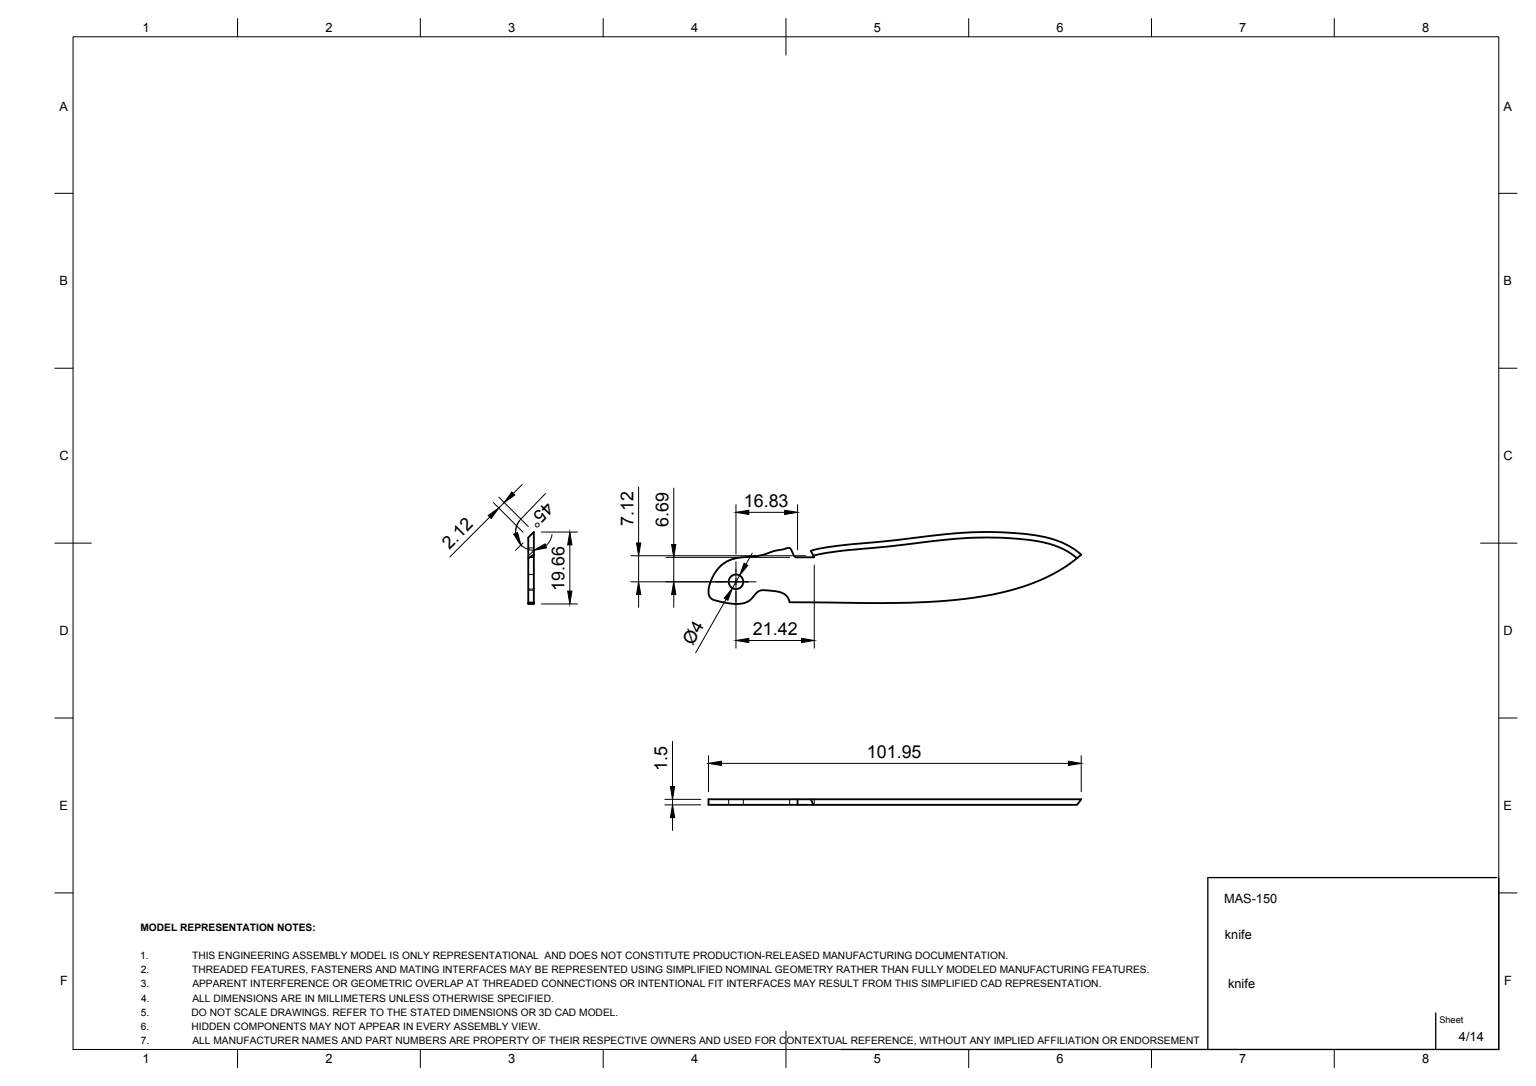
ISO-10303-21;
HEADER;
/* Generated by software containing ST-Developer
 * from STEP Tools, Inc. (www.steptools.com) 
 */

FILE_DESCRIPTION(
/* description */ ('STEP AP203'),
/* implementation_level */ '2;1');

FILE_NAME(
/* name */ 'knife.step',
/* time_stamp */ '2026-11-08T21:40:52-08:00',
/* author */ (''),
/* organization */ (''),
/* preprocessor_version */ 'ST-DEVELOPER v20.2',
/* originating_system */ 'Autodesk Translation Framework v15.17.0.0',
/* authorisation */ '');

FILE_SCHEMA (('AUTOMOTIVE_DESIGN { 1 0 10303 214 3 1 1 }'));
ENDSEC;

DATA;
#10=MECHANICAL_DESIGN_GEOMETRIC_PRESENTATION_REPRESENTATION('',(#184),#12137);
#81=B_SPLINE_CURVE_WITH_KNOTS('',3,(#2753,#2754,#2755,#2756,#2757,#2758,
#2759,#2760,#2761,#2762,#2763,#2764),.UNSPECIFIED.,.F.,.F.,(4,1,1,1,1,1,
1,1,1,4),(0.692277335272932,0.69714998216664,0.713058394872634,0.723664003343296,
0.736358399716042,0.759577826910316,0.780092040409136,0.810242072545427,
0.901462701662728,0.958125874426747),.UNSPECIFIED.);
#82=B_SPLINE_CURVE_WITH_KNOTS('',3,(#2768,#2769,#2770,#2771,#2772,#2773,
#2774,#2775,#2776,#2777,#2778,#2779),.UNSPECIFIED.,.F.,.F.,(4,1,1,1,1,1,
1,1,1,4),(0.692277335272932,0.69714998216664,0.713058394872634,0.723664003343296,
0.736358399716042,0.759577826910316,0.780092040409136,0.810242072545427,
0.901462701662728,0.958125874426747),.UNSPECIFIED.);
#83=B_SPLINE_CURVE_WITH_KNOTS('',3,(#2794,#2795,#2796,#2797,#2798,#2799),
 .UNSPECIFIED.,.F.,.F.,(4,1,1,4),(0.,0.587279823509184,0.66516934088919,
1.),.UNSPECIFIED.);
#84=B_SPLINE_CURVE_WITH_KNOTS('',3,(#2802,#2803,#2804,#2805,#2806,#2807),
 .UNSPECIFIED.,.F.,.F.,(4,1,1,4),(0.,0.587279823509184,0.66516934088919,
1.),.UNSPECIFIED.);
#85=B_SPLINE_CURVE_WITH_KNOTS('',3,(#2823,#2824,#2825,#2826,#2827,#2828,
#2829),.UNSPECIFIED.,.F.,.F.,(4,1,1,1,4),(0.,0.0866729836098282,0.459841695939614,
0.649673299675604,0.845208562818702),.UNSPECIFIED.);
#86=B_SPLINE_CURVE_WITH_KNOTS('',3,(#2831,#2832,#2833,#2834,#2835,#2836,
#2837),.UNSPECIFIED.,.F.,.F.,(4,3,4),(1.35324872955864E-8,0.631650088317911,
1.),.UNSPECIFIED.);
#87=B_SPLINE_CURVE_WITH_KNOTS('',3,(#2838,#2839,#2840,#2841,#2842,#2843,
#2844),.UNSPECIFIED.,.F.,.F.,(4,1,1,1,4),(0.,0.0866729836098282,0.459841695939614,
0.649673299675604,0.829767002127536),.UNSPECIFIED.);
#88=B_SPLINE_CURVE_WITH_KNOTS('',3,(#2847,#2848,#2849,#2850,#2851,#2852,
#2853,#2854,#2855,#2856,#2857,#2858,#2859,#2860,#2861,#2862,#2863,#2864,
#2865,#2866,#2867,#2868,#2869,#2870,#2871,#2872,#2873,#2874,#2875,#2876,
#2877,#2878,#2879,#2880,#2881,#2882,#2883,#2884,#2885,#2886,#2887,#2888,
#2889,#2890,#2891,#2892,#2893,#2894,#2895,#2896,#2897,#2898,#2899,#2900,
#2901,#2902,#2903,#2904,#2905,#2906,#2907,#2908,#2909,#2910,#2911,#2912,
#2913,#2914,#2915,#2916,#2917,#2918,#2919,#2920,#2921,#2922,#2923,#2924,
#2925,#2926,#2927,#2928,#2929,#2930,#2931,#2932,#2933,#2934,#2935,#2936,
#2937,#2938,#2939,#2940,#2941,#2942,#2943,#2944,#2945,#2946,#2947,#2948,
#2949,#2950,#2951,#2952,#2953,#2954,#2955,#2956,#2957,#2958,#2959,#2960,
#2961,#2962,#2963,#2964,#2965,#2966,#2967,#2968,#2969,#2970,#2971,#2972,
#2973,#2974,#2975,#2976,#2977,#2978,#2979,#2980,#2981,#2982,#2983,#2984,
#2985,#2986,#2987,#2988,#2989,#2990,#2991,#2992,#2993,#2994,#2995,#2996,
#2997,#2998,#2999,#3000,#3001,#3002,#3003,#3004,#3005,#3006,#3007,#3008,
#3009,#3010,#3011,#3012,#3013,#3014,#3015,#3016,#3017,#3018,#3019,#3020,
#3021,#3022,#3023,#3024,#3025,#3026,#3027,#3028,#3029,#3030,#3031,#3032,
#3033,#3034,#3035,#3036,#3037,#3038,#3039,#3040,#3041,#3042,#3043,#3044,
#3045,#3046,#3047,#3048,#3049,#3050,#3051,#3052,#3053,#3054,#3055,#3056,
#3057,#3058,#3059,#3060,#3061,#3062,#3063,#3064,#3065,#3066,#3067,#3068,
#3069,#3070,#3071,#3072,#3073,#3074,#3075,#3076,#3077,#3078,#3079,#3080,
#3081,#3082,#3083,#3084,#3085,#3086,#3087,#3088,#3089,#3090,#3091,#3092,
#3093,#3094,#3095,#3096,#3097,#3098,#3099,#3100,#3101,#3102,#3103,#3104,
#3105,#3106,#3107,#3108,#3109,#3110,#3111,#3112,#3113,#3114,#3115,#3116,
#3117,#3118,#3119,#3120,#3121,#3122,#3123,#3124,#3125,#3126,#3127,#3128,
#3129,#3130,#3131,#3132,#3133,#3134,#3135,#3136,#3137,#3138,#3139,#3140,
#3141,#3142,#3143,#3144,#3145,#3146,#3147,#3148,#3149,#3150,#3151,#3152,
#3153,#3154,#3155,#3156,#3157,#3158,#3159,#3160,#3161,#3162,#3163,#3164,
#3165,#3166,#3167,#3168,#3169,#3170,#3171,#3172,#3173,#3174,#3175,#3176,
#3177),.UNSPECIFIED.,.F.,.F.,(4,3,3,3,3,3,3,3,3,3,3,3,3,3,3,3,3,3,3,3,3,
3,3,3,3,3,3,3,3,3,3,3,3,3,3,3,3,3,3,3,3,3,3,3,3,3,3,3,3,3,3,3,3,3,3,3,3,
3,3,3,3,3,3,3,3,3,3,3,3,3,3,3,3,3,3,3,3,3,3,3,3,3,3,3,3,3,3,3,3,3,3,3,3,
3,3,3,3,3,3,3,3,3,3,3,3,3,3,3,3,3,4),(1.00000005226737E-6,0.00728562366971475,
0.0234463959847306,0.0557978953419903,0.0881792075542466,0.120578085908497,
0.199435146924132,0.250102975200852,0.332264327598246,0.378931394146745,
0.442710847956035,0.458655711408358,0.465225430544162,0.470485225689555,
0.506490301765326,0.587406978409983,0.63447750239409,0.698713581314966,
0.762996361968068,0.827238553299382,0.891353412993002,0.919885897936909,
0.925235738863892,0.927910373024815,0.929197830974231,0.93032386627772,
0.965310836068324,1.00172317218786,1.00548335276863,1.0439300169432,1.08610137935927,
1.14148474424288,1.17398141008201,1.20363917088317,1.23143564581068,1.25060619127644,
1.27597878060136,1.29260925110888,1.33079359731686,1.3485547264891,1.3496219232794,
1.35038687476659,1.36631585566134,1.43886146909154,1.48931728875302,1.51524396218266,
1.57648663203031,1.5962584262802,1.66704233666681,1.6830136697589,1.74924243686783,
1.77713875907306,1.81979916869953,1.82771178722931,1.87226124160844,1.8812062035948,
1.92683921666331,1.96328819238212,1.98151268024153,1.99062492417124,1.99518104613609,
1.99809663447909,1.99973716810094,2.11425198948044,2.25593468219522,2.3831520244116,
2.49139452866391,2.51036936662798,2.54228741890446,2.56622595811182,2.57160131643996,
2.57333509499776,2.63448414790964,2.63804157573391,2.70877992194418,2.77951826815446,
2.85750983652355,2.92223429974548,2.94135846274582,3.00435550993043,3.07158275602607,
3.13078242154972,3.20465260936858,3.28573698285387,3.35844860482519,3.42587818692828,
3.4764503735056,3.48117348962947,3.48410509148297,3.62816693323756,3.7643950388047,
3.88405944557012,3.90062314437185,4.00766553231559,4.10852611031876,4.17975199447887,
4.27429663966353,4.32614318790147,4.41732790628579,4.48050879966944,4.56192648809965,
4.60400180805684,4.64714550046042,4.69150379518099,4.73725365207584,4.7884515645196,
4.83385532714358,4.88768324231123,4.93951305213049,4.99975507375154,5.03337263030683),
 .UNSPECIFIED.);
#89=B_SPLINE_CURVE_WITH_KNOTS('',3,(#3186,#3187,#3188,#3189,#3190,#3191,
#3192,#3193,#3194,#3195,#3196,#3197,#3198,#3199,#3200,#3201,#3202,#3203,
#3204,#3205,#3206,#3207,#3208,#3209,#3210,#3211,#3212,#3213,#3214,#3215,
#3216,#3217,#3218,#3219,#3220,#3221,#3222,#3223,#3224,#3225,#3226,#3227,
#3228,#3229,#3230,#3231,#3232,#3233,#3234,#3235,#3236,#3237,#3238,#3239,
#3240,#3241,#3242,#3243,#3244,#3245,#3246,#3247,#3248,#3249,#3250,#3251,
#3252,#3253,#3254,#3255,#3256,#3257,#3258,#3259,#3260,#3261,#3262,#3263,
#3264,#3265,#3266,#3267,#3268,#3269,#3270,#3271,#3272,#3273,#3274,#3275,
#3276,#3277,#3278,#3279,#3280,#3281,#3282,#3283,#3284,#3285,#3286,#3287,
#3288,#3289,#3290,#3291,#3292,#3293,#3294,#3295,#3296),.UNSPECIFIED.,.F.,
 .F.,(4,2,2,2,2,1,2,2,2,2,2,2,2,2,2,2,2,2,2,2,2,2,2,2,2,2,2,2,2,2,2,2,2,
2,2,2,2,2,2,2,2,2,2,2,2,2,2,2,2,2,2,2,2,2,2,4),(0.,0.000220711532429116,
0.000489265959006191,0.00102637481216034,0.00156348366531445,0.0026377013716227,
0.003711919077931,0.00586035449054751,0.0101572253157805,0.0144540961410136,
0.0187509669662467,0.0359384502671788,0.0531259335681111,0.0703134168690433,
0.0875009001699755,0.0960946418204416,0.104688383470908,0.113282125121374,
0.12187586677184,0.139063350072772,0.156250833373704,0.190625799975569,
0.207813283276501,0.225000766577433,0.242188249878365,0.259375733179298,
0.293750699781162,0.328125666383026,0.362500632984891,0.396875599586755,
0.43125056618862,0.448438049489552,0.465625532790484,0.500000499392348,
0.568750432596077,0.637500365799806,0.67187533240167,0.706250299003535,
0.723437782304467,0.740625265605399,0.775000232207264,0.809375198809128,
0.843750165410992,0.878125132012857,0.912500098614721,0.929687581915653,
0.946875065216586,0.955468806867052,0.959765677692285,0.964062548517518,
0.968359419342751,0.972656290167984,0.98125003181845,0.989843773468916,
0.998437515119382,0.999999994546672),.UNSPECIFIED.);
#90=B_SPLINE_CURVE_WITH_KNOTS('',3,(#3298,#3299,#3300,#3301,#3302,#3303),
 .UNSPECIFIED.,.F.,.F.,(4,2,4),(9.43755849736976E-11,0.103884415747993,
0.213656518400476),.UNSPECIFIED.);
#138=B_SPLINE_SURFACE_WITH_KNOTS('',3,1,((#2727,#2728),(#2729,#2730),(#2731,
#2732),(#2733,#2734),(#2735,#2736),(#2737,#2738),(#2739,#2740),(#2741,#2742),
(#2743,#2744),(#2745,#2746),(#2747,#2748),(#2749,#2750)),.UNSPECIFIED.,
 .F.,.F.,.F.,(4,1,1,1,1,1,1,1,1,4),(2,2),(0.692277335272932,0.69714998216664,
0.713058394872634,0.723664003343296,0.736358399716042,0.759577826910316,
0.780092040409136,0.810242072545427,0.901462701662728,0.958125874426747),
(0.,0.216),.UNSPECIFIED.);
#139=B_SPLINE_SURFACE_WITH_KNOTS('',3,1,((#2781,#2782),(#2783,#2784),(#2785,
#2786),(#2787,#2788),(#2789,#2790),(#2791,#2792)),.UNSPECIFIED.,.F.,.F.,
 .F.,(4,1,1,4),(2,2),(0.,0.587279823509184,0.66516934088919,1.),(0.,0.216),
 .UNSPECIFIED.);
#140=B_SPLINE_SURFACE_WITH_KNOTS('',3,1,((#2808,#2809),(#2810,#2811),(#2812,
#2813),(#2814,#2815),(#2816,#2817),(#2818,#2819),(#2820,#2821)),
 .UNSPECIFIED.,.F.,.F.,.F.,(4,1,1,1,4),(2,2),(0.,0.0866729836098282,0.459841695939614,
0.649673299675604,0.845208563176808),(0.,0.216000000047327),
 .UNSPECIFIED.);
#141=B_SPLINE_SURFACE_WITH_KNOTS('',1,3,((#3306,#3307,#3308,#3309,#3310,
#3311,#3312,#3313,#3314,#3315,#3316,#3317,#3318,#3319,#3320,#3321,#3322,
#3323,#3324,#3325,#3326,#3327,#3328,#3329,#3330,#3331,#3332,#3333,#3334,
#3335,#3336,#3337,#3338,#3339,#3340,#3341,#3342,#3343,#3344,#3345,#3346,
#3347,#3348,#3349,#3350,#3351,#3352,#3353,#3354,#3355,#3356,#3357,#3358,
#3359,#3360,#3361,#3362,#3363,#3364,#3365,#3366,#3367,#3368,#3369,#3370,
#3371,#3372,#3373,#3374,#3375,#3376,#3377,#3378,#3379,#3380,#3381,#3382,
#3383,#3384,#3385,#3386,#3387,#3388,#3389,#3390,#3391,#3392,#3393,#3394,
#3395,#3396,#3397,#3398,#3399,#3400,#3401,#3402,#3403,#3404,#3405,#3406,
#3407,#3408,#3409,#3410,#3411,#3412,#3413,#3414,#3415,#3416,#3417,#3418,
#3419,#3420,#3421,#3422,#3423,#3424,#3425,#3426,#3427,#3428,#3429,#3430,
#3431,#3432,#3433,#3434,#3435,#3436,#3437,#3438,#3439,#3440,#3441,#3442,
#3443,#3444,#3445,#3446,#3447,#3448,#3449,#3450,#3451,#3452,#3453,#3454,
#3455,#3456,#3457,#3458,#3459,#3460,#3461),(#3462,#3463,#3464,#3465,#3466,
#3467,#3468,#3469,#3470,#3471,#3472,#3473,#3474,#3475,#3476,#3477,#3478,
#3479,#3480,#3481,#3482,#3483,#3484,#3485,#3486,#3487,#3488,#3489,#3490,
#3491,#3492,#3493,#3494,#3495,#3496,#3497,#3498,#3499,#3500,#3501,#3502,
#3503,#3504,#3505,#3506,#3507,#3508,#3509,#3510,#3511,#3512,#3513,#3514,
#3515,#3516,#3517,#3518,#3519,#3520,#3521,#3522,#3523,#3524,#3525,#3526,
#3527,#3528,#3529,#3530,#3531,#3532,#3533,#3534,#3535,#3536,#3537,#3538,
#3539,#3540,#3541,#3542,#3543,#3544,#3545,#3546,#3547,#3548,#3549,#3550,
#3551,#3552,#3553,#3554,#3555,#3556,#3557,#3558,#3559,#3560,#3561,#3562,
#3563,#3564,#3565,#3566,#3567,#3568,#3569,#3570,#3571,#3572,#3573,#3574,
#3575,#3576,#3577,#3578,#3579,#3580,#3581,#3582,#3583,#3584,#3585,#3586,
#3587,#3588,#3589,#3590,#3591,#3592,#3593,#3594,#3595,#3596,#3597,#3598,
#3599,#3600,#3601,#3602,#3603,#3604,#3605,#3606,#3607,#3608,#3609,#3610,
#3611,#3612,#3613,#3614,#3615,#3616,#3617)),.UNSPECIFIED.,.F.,.F.,.F.,(2,
2),(4,2,2,2,2,2,2,2,2,2,2,2,2,2,2,2,2,2,2,2,2,2,2,2,2,2,2,2,2,2,2,2,2,2,
2,2,2,2,2,2,2,2,2,2,2,2,2,2,2,2,2,2,2,2,2,2,2,2,2,2,2,2,2,2,2,2,2,2,2,2,
2,2,2,2,2,2,2,4),(-2.82979241385037E-6,1.00000282979242),(0.0211247699785431,
0.0224166474384851,0.023062586168456,0.023708524898427,0.0240314942634125,
0.024354463628398,0.0246774329933834,0.0247581753346298,0.024798546505253,
0.0248389176758762,0.0248591032611878,0.0248792888464994,0.0248994744318109,
0.0249196600171225,0.0249600311877457,0.0250004023583689,0.0250811446996153,
0.0251618870408617,0.0253233717233544,0.0256463410883399,0.0259693104533254,
0.0262922798183108,0.0275841572782528,0.0288760347381947,0.0301679121981366,
0.0314597896580785,0.0321057283880495,0.0327516671180205,0.0333976058479914,
0.0340435445779624,0.0353354220379043,0.0366272994978462,0.0392110544177301,
0.040502931877672,0.0417948093376139,0.0430866867975558,0.0443785642574978,
0.0469623191773816,0.0495460740972655,0.0521298290171493,0.0547135839370332,
0.057297338856917,0.0585892163168589,0.0598810937768009,0.0624648486966847,
0.0676323585364524,0.0727998683762201,0.0753836232961039,0.0779673782159878,
0.0792592556759297,0.0805511331358716,0.0831348880557555,0.0857186429756393,
0.0883023978955232,0.090886152815407,0.0934699077352909,0.0947617851952328,
0.0960536626551747,0.0966996013851457,0.0970225707501312,0.0973455401151166,
0.0976685094801021,0.0979914788450876,0.0986374175750586,0.0992833563050295,
0.0999292950350005,0.100575233764971,0.101221172494942,0.101544141859928,
0.101867111224913,0.102028595907406,0.102190080589899,0.102270822931145,
0.102351565272392,0.102513049954884,0.10283601931987,0.103158988684855,
0.103804927414826),.UNSPECIFIED.);
#162=SHAPE_REPRESENTATION_RELATIONSHIP('SRR','None',#12185,#173);
#173=ADVANCED_BREP_SHAPE_REPRESENTATION('',(#195),#12126);
#184=STYLED_ITEM('',(#12253),#195);
#195=MANIFOLD_SOLID_BREP('Body1',#1829);
#209=FACE_BOUND('',#623,.T.);
#210=FACE_BOUND('',#625,.T.);
#236=PLANE('',#2001);
#237=PLANE('',#2002);
#238=PLANE('',#2003);
#239=PLANE('',#2004);
#288=LINE('',#2725,#382);
#289=LINE('',#2766,#383);
#290=LINE('',#2780,#384);
#291=LINE('',#2801,#385);
#292=LINE('',#3179,#386);
#293=LINE('',#3180,#387);
#294=LINE('',#3183,#388);
#295=LINE('',#3185,#389);
#296=LINE('',#3304,#390);
#382=VECTOR('',#2250,2.);
#383=VECTOR('',#2253,1000.);
#384=VECTOR('',#2254,1000.);
#385=VECTOR('',#2255,1000.);
#386=VECTOR('',#2258,1000.);
#387=VECTOR('',#2259,1000.);
#388=VECTOR('',#2262,1000.);
#389=VECTOR('',#2263,1000.);
#390=VECTOR('',#2266,1000.);
#470=CYLINDRICAL_SURFACE('',#1998,2.);
#504=FACE_OUTER_BOUND('',#618,.T.);
#505=FACE_OUTER_BOUND('',#619,.T.);
#506=FACE_OUTER_BOUND('',#620,.T.);
#507=FACE_OUTER_BOUND('',#621,.T.);
#508=FACE_OUTER_BOUND('',#622,.T.);
#509=FACE_OUTER_BOUND('',#624,.T.);
#510=FACE_OUTER_BOUND('',#626,.T.);
#511=FACE_OUTER_BOUND('',#627,.T.);
#512=FACE_OUTER_BOUND('',#628,.T.);
#618=EDGE_LOOP('',(#1287,#1288,#1289,#1290));
#619=EDGE_LOOP('',(#1291,#1292,#1293,#1294));
#620=EDGE_LOOP('',(#1295,#1296,#1297,#1298));
#621=EDGE_LOOP('',(#1299,#1300,#1301,#1302));
#622=EDGE_LOOP('',(#1303,#1304,#1305,#1306,#1307,#1308));
#623=EDGE_LOOP('',(#1309));
#624=EDGE_LOOP('',(#1310,#1311,#1312,#1313,#1314,#1315));
#625=EDGE_LOOP('',(#1316));
#626=EDGE_LOOP('',(#1317,#1318,#1319,#1320));
#627=EDGE_LOOP('',(#1321,#1322,#1323,#1324));
#628=EDGE_LOOP('',(#1325,#1326,#1327,#1328));
#757=CIRCLE('',#1999,2.);
#758=CIRCLE('',#2000,2.);
#844=VERTEX_POINT('',#2722);
#845=VERTEX_POINT('',#2724);
#846=VERTEX_POINT('',#2751);
#847=VERTEX_POINT('',#2752);
#848=VERTEX_POINT('',#2765);
#849=VERTEX_POINT('',#2767);
#850=VERTEX_POINT('',#2793);
#851=VERTEX_POINT('',#2800);
#852=VERTEX_POINT('',#2822);
#853=VERTEX_POINT('',#2830);
#854=VERTEX_POINT('',#2846);
#855=VERTEX_POINT('',#3178);
#856=VERTEX_POINT('',#3182);
#857=VERTEX_POINT('',#3184);
#1013=EDGE_CURVE('',#844,#844,#757,.T.);
#1014=EDGE_CURVE('',#844,#845,#288,.T.);
#1015=EDGE_CURVE('',#845,#845,#758,.T.);
#1016=EDGE_CURVE('',#846,#847,#81,.T.);
#1017=EDGE_CURVE('',#848,#846,#289,.T.);
#1018=EDGE_CURVE('',#848,#849,#82,.T.);
#1019=EDGE_CURVE('',#847,#849,#290,.T.);
#1020=EDGE_CURVE('',#849,#850,#83,.T.);
#1021=EDGE_CURVE('',#851,#850,#291,.T.);
#1022=EDGE_CURVE('',#847,#851,#84,.T.);
#1023=EDGE_CURVE('',#850,#852,#85,.T.);
#1024=EDGE_CURVE('',#852,#853,#86,.T.);
#1025=EDGE_CURVE('',#851,#853,#87,.T.);
#1026=EDGE_CURVE('',#853,#854,#88,.T.);
#1027=EDGE_CURVE('',#855,#854,#292,.T.);
#1028=EDGE_CURVE('',#846,#855,#293,.T.);
#1029=EDGE_CURVE('',#848,#856,#294,.T.);
#1030=EDGE_CURVE('',#856,#857,#295,.T.);
#1031=EDGE_CURVE('',#852,#857,#89,.T.);
#1032=EDGE_CURVE('',#854,#857,#90,.T.);
#1033=EDGE_CURVE('',#856,#855,#296,.T.);
#1287=ORIENTED_EDGE('',*,*,#1013,.T.);
#1288=ORIENTED_EDGE('',*,*,#1014,.T.);
#1289=ORIENTED_EDGE('',*,*,#1015,.T.);
#1290=ORIENTED_EDGE('',*,*,#1014,.F.);
#1291=ORIENTED_EDGE('',*,*,#1016,.F.);
#1292=ORIENTED_EDGE('',*,*,#1017,.F.);
#1293=ORIENTED_EDGE('',*,*,#1018,.T.);
#1294=ORIENTED_EDGE('',*,*,#1019,.F.);
#1295=ORIENTED_EDGE('',*,*,#1020,.T.);
#1296=ORIENTED_EDGE('',*,*,#1021,.F.);
#1297=ORIENTED_EDGE('',*,*,#1022,.F.);
#1298=ORIENTED_EDGE('',*,*,#1019,.T.);
#1299=ORIENTED_EDGE('',*,*,#1023,.T.);
#1300=ORIENTED_EDGE('',*,*,#1024,.T.);
#1301=ORIENTED_EDGE('',*,*,#1025,.F.);
#1302=ORIENTED_EDGE('',*,*,#1021,.T.);
#1303=ORIENTED_EDGE('',*,*,#1025,.T.);
#1304=ORIENTED_EDGE('',*,*,#1026,.T.);
#1305=ORIENTED_EDGE('',*,*,#1027,.F.);
#1306=ORIENTED_EDGE('',*,*,#1028,.F.);
#1307=ORIENTED_EDGE('',*,*,#1016,.T.);
#1308=ORIENTED_EDGE('',*,*,#1022,.T.);
#1309=ORIENTED_EDGE('',*,*,#1015,.F.);
#1310=ORIENTED_EDGE('',*,*,#1029,.T.);
#1311=ORIENTED_EDGE('',*,*,#1030,.T.);
#1312=ORIENTED_EDGE('',*,*,#1031,.F.);
#1313=ORIENTED_EDGE('',*,*,#1023,.F.);
#1314=ORIENTED_EDGE('',*,*,#1020,.F.);
#1315=ORIENTED_EDGE('',*,*,#1018,.F.);
#1316=ORIENTED_EDGE('',*,*,#1013,.F.);
#1317=ORIENTED_EDGE('',*,*,#1027,.T.);
#1318=ORIENTED_EDGE('',*,*,#1032,.T.);
#1319=ORIENTED_EDGE('',*,*,#1030,.F.);
#1320=ORIENTED_EDGE('',*,*,#1033,.T.);
#1321=ORIENTED_EDGE('',*,*,#1028,.T.);
#1322=ORIENTED_EDGE('',*,*,#1033,.F.);
#1323=ORIENTED_EDGE('',*,*,#1029,.F.);
#1324=ORIENTED_EDGE('',*,*,#1017,.T.);
#1325=ORIENTED_EDGE('',*,*,#1024,.F.);
#1326=ORIENTED_EDGE('',*,*,#1031,.T.);
#1327=ORIENTED_EDGE('',*,*,#1032,.F.);
#1328=ORIENTED_EDGE('',*,*,#1026,.F.);
#1732=ADVANCED_FACE('',(#504),#470,.F.);
#1733=ADVANCED_FACE('',(#505),#138,.F.);
#1734=ADVANCED_FACE('',(#506),#139,.F.);
#1735=ADVANCED_FACE('',(#507),#140,.F.);
#1736=ADVANCED_FACE('',(#508,#209),#236,.F.);
#1737=ADVANCED_FACE('',(#509,#210),#237,.T.);
#1738=ADVANCED_FACE('',(#510),#238,.F.);
#1739=ADVANCED_FACE('',(#511),#239,.F.);
#1740=ADVANCED_FACE('',(#512),#141,.T.);
#1829=CLOSED_SHELL('',(#1732,#1733,#1734,#1735,#1736,#1737,#1738,#1739,
#1740));
#1997=AXIS2_PLACEMENT_3D('',#2720,#2244,#2245);
#1998=AXIS2_PLACEMENT_3D('',#2721,#2246,#2247);
#1999=AXIS2_PLACEMENT_3D('',#2723,#2248,#2249);
#2000=AXIS2_PLACEMENT_3D('',#2726,#2251,#2252);
#2001=AXIS2_PLACEMENT_3D('',#2845,#2256,#2257);
#2002=AXIS2_PLACEMENT_3D('',#3181,#2260,#2261);
#2003=AXIS2_PLACEMENT_3D('',#3297,#2264,#2265);
#2004=AXIS2_PLACEMENT_3D('',#3305,#2267,#2268);
#2244=DIRECTION('axis',(0.,0.,1.));
#2245=DIRECTION('refdir',(1.,0.,0.));
#2246=DIRECTION('center_axis',(0.,1.,0.));
#2247=DIRECTION('ref_axis',(0.,0.,1.));
#2248=DIRECTION('center_axis',(0.,-1.,0.));
#2249=DIRECTION('ref_axis',(0.,0.,-1.));
#2250=DIRECTION('',(0.,1.,0.));
#2251=DIRECTION('center_axis',(0.,1.,0.));
#2252=DIRECTION('ref_axis',(0.,0.,1.));
#2253=DIRECTION('',(0.,1.,0.));
#2254=DIRECTION('',(0.,-1.,0.));
#2255=DIRECTION('',(0.,-1.,0.));
#2256=DIRECTION('center_axis',(0.,-1.,0.));
#2257=DIRECTION('ref_axis',(0.,0.,-1.));
#2258=DIRECTION('',(0.472839131639098,0.,0.881148770407576));
#2259=DIRECTION('',(-1.,0.,0.));
#2260=DIRECTION('center_axis',(0.,-1.,0.));
#2261=DIRECTION('ref_axis',(0.,0.,-1.));
#2262=DIRECTION('',(-1.,0.,0.));
#2263=DIRECTION('',(0.472839131639098,0.,0.881148770407576));
#2264=DIRECTION('center_axis',(-0.881148770407576,0.,0.472839131639098));
#2265=DIRECTION('ref_axis',(0.472839131639098,0.,0.881148770407576));
#2266=DIRECTION('',(0.,1.,0.));
#2267=DIRECTION('center_axis',(0.,0.,-1.));
#2268=DIRECTION('ref_axis',(-1.,0.,0.));
#2720=CARTESIAN_POINT('',(0.,0.,0.));
#2721=CARTESIAN_POINT('Origin',(42.7532306583709,-0.000750036417118335,
-2.95713890544537));
#2722=CARTESIAN_POINT('',(42.7532306583709,0.,-4.95713890544537));
#2723=CARTESIAN_POINT('Origin',(42.7532306583709,0.,-2.95713890544537));
#2724=CARTESIAN_POINT('',(42.7532306583709,1.5,-4.95713890544537));
#2725=CARTESIAN_POINT('',(42.7532306583709,-0.000750036417118335,-4.95713890544537));
#2726=CARTESIAN_POINT('Origin',(42.7532306583709,1.5,-2.95713890544537));
#2727=CARTESIAN_POINT('Ctrl Pts',(25.9188618862632,1.5,3.73655812708952));
#2728=CARTESIAN_POINT('Ctrl Pts',(25.9188618862632,-0.66,3.73655812708952));
#2729=CARTESIAN_POINT('Ctrl Pts',(26.0838087555079,1.5,3.69528174729993));
#2730=CARTESIAN_POINT('Ctrl Pts',(26.0838087555079,-0.66,3.69528174729993));
#2731=CARTESIAN_POINT('Ctrl Pts',(26.7414333467756,1.5,3.66889628312799));
#2732=CARTESIAN_POINT('Ctrl Pts',(26.7414333467756,-0.66,3.66889628312799));
#2733=CARTESIAN_POINT('Ctrl Pts',(27.3011855299882,1.5,5.05266376239426));
#2734=CARTESIAN_POINT('Ctrl Pts',(27.3011855299882,-0.66,5.05266376239426));
#2735=CARTESIAN_POINT('Ctrl Pts',(27.9697213442539,1.5,6.64187212001263));
#2736=CARTESIAN_POINT('Ctrl Pts',(27.9697213442539,-0.66,6.64187212001263));
#2737=CARTESIAN_POINT('Ctrl Pts',(30.0035737390622,1.5,5.70550320798981));
#2738=CARTESIAN_POINT('Ctrl Pts',(30.0035737390622,-0.66,5.70550320798981));
#2739=CARTESIAN_POINT('Ctrl Pts',(31.8783416154944,1.5,5.75245772223251));
#2740=CARTESIAN_POINT('Ctrl Pts',(31.8783416154944,-0.66,5.75245772223251));
#2741=CARTESIAN_POINT('Ctrl Pts',(35.1844604255421,1.5,4.32025211416494));
#2742=CARTESIAN_POINT('Ctrl Pts',(35.1844604255421,-0.66,4.32025211416494));
#2743=CARTESIAN_POINT('Ctrl Pts',(40.192401529867,1.5,3.55204841770967));
#2744=CARTESIAN_POINT('Ctrl Pts',(40.192401529867,-0.66,3.55204841770967));
#2745=CARTESIAN_POINT('Ctrl Pts',(47.9284527442042,1.5,4.14235365515584));
#2746=CARTESIAN_POINT('Ctrl Pts',(47.9284527442042,-0.66,4.14235365515584));
#2747=CARTESIAN_POINT('Ctrl Pts',(51.435120996177,1.5,-7.206342921025));
#2748=CARTESIAN_POINT('Ctrl Pts',(51.435120996177,-0.66,-7.206342921025));
#2749=CARTESIAN_POINT('Ctrl Pts',(48.7532306583708,1.5,-7.95408926393385));
#2750=CARTESIAN_POINT('Ctrl Pts',(48.7532306583708,-0.66,-7.95408926393385));
#2751=CARTESIAN_POINT('',(25.9188618861119,1.5,3.73655812712738));
#2752=CARTESIAN_POINT('',(48.7532306583709,1.5,-7.95408926393383));
#2753=CARTESIAN_POINT('Ctrl Pts',(25.9188618862632,1.5,3.73655812708952));
#2754=CARTESIAN_POINT('Ctrl Pts',(26.0838087555079,1.5,3.69528174729993));
#2755=CARTESIAN_POINT('Ctrl Pts',(26.7414333467756,1.5,3.66889628312799));
#2756=CARTESIAN_POINT('Ctrl Pts',(27.3011855299882,1.5,5.05266376239426));
#2757=CARTESIAN_POINT('Ctrl Pts',(27.9697213442539,1.5,6.64187212001263));
#2758=CARTESIAN_POINT('Ctrl Pts',(30.0035737390622,1.5,5.70550320798981));
#2759=CARTESIAN_POINT('Ctrl Pts',(31.8783416154944,1.5,5.75245772223251));
#2760=CARTESIAN_POINT('Ctrl Pts',(35.1844604255421,1.5,4.32025211416494));
#2761=CARTESIAN_POINT('Ctrl Pts',(40.192401529867,1.5,3.55204841770967));
#2762=CARTESIAN_POINT('Ctrl Pts',(47.9284527442042,1.5,4.14235365515584));
#2763=CARTESIAN_POINT('Ctrl Pts',(51.435120996177,1.5,-7.206342921025));
#2764=CARTESIAN_POINT('Ctrl Pts',(48.7532306583708,1.5,-7.95408926393385));
#2765=CARTESIAN_POINT('',(25.9188618861119,0.,3.73655812712738));
#2766=CARTESIAN_POINT('',(25.9188618861119,0.,3.73655812712738));
#2767=CARTESIAN_POINT('',(48.7532306583709,0.,-7.95408926393383));
#2768=CARTESIAN_POINT('Ctrl Pts',(25.9188618862632,0.,3.73655812708952));
#2769=CARTESIAN_POINT('Ctrl Pts',(26.0838087555079,0.,3.69528174729993));
#2770=CARTESIAN_POINT('Ctrl Pts',(26.7414333467756,0.,3.66889628312799));
#2771=CARTESIAN_POINT('Ctrl Pts',(27.3011855299882,0.,5.05266376239426));
#2772=CARTESIAN_POINT('Ctrl Pts',(27.9697213442539,0.,6.64187212001263));
#2773=CARTESIAN_POINT('Ctrl Pts',(30.0035737390622,0.,5.70550320798981));
#2774=CARTESIAN_POINT('Ctrl Pts',(31.8783416154944,0.,5.75245772223251));
#2775=CARTESIAN_POINT('Ctrl Pts',(35.1844604255421,0.,4.32025211416494));
#2776=CARTESIAN_POINT('Ctrl Pts',(40.192401529867,0.,3.55204841770967));
#2777=CARTESIAN_POINT('Ctrl Pts',(47.9284527442042,0.,4.14235365515584));
#2778=CARTESIAN_POINT('Ctrl Pts',(51.435120996177,0.,-7.206342921025));
#2779=CARTESIAN_POINT('Ctrl Pts',(48.7532306583708,0.,-7.95408926393385));
#2780=CARTESIAN_POINT('',(48.7532306583709,1.5,-7.95408926393383));
#2781=CARTESIAN_POINT('Ctrl Pts',(48.7532306583709,1.5,-7.95408926393383));
#2782=CARTESIAN_POINT('Ctrl Pts',(48.7532306583709,-0.66,-7.95408926393383));
#2783=CARTESIAN_POINT('Ctrl Pts',(36.6068452277914,1.5,-11.3406614728137));
#2784=CARTESIAN_POINT('Ctrl Pts',(36.6068452277914,-0.66,-11.3406614728137));
#2785=CARTESIAN_POINT('Ctrl Pts',(39.4535021242481,1.5,-4.7454968822424));
#2786=CARTESIAN_POINT('Ctrl Pts',(39.4535021242481,-0.66,-4.7454968822424));
#2787=CARTESIAN_POINT('Ctrl Pts',(31.9355686583357,1.5,-5.55619061474896));
#2788=CARTESIAN_POINT('Ctrl Pts',(31.9355686583357,-0.66,-5.55619061474896));
#2789=CARTESIAN_POINT('Ctrl Pts',(28.7242328419571,1.5,-5.63921626360694));
#2790=CARTESIAN_POINT('Ctrl Pts',(28.7242328419571,-0.66,-5.63921626360694));
#2791=CARTESIAN_POINT('Ctrl Pts',(28.0628515535919,1.5,-8.54333666903048));
#2792=CARTESIAN_POINT('Ctrl Pts',(28.0628515535919,-0.66,-8.54333666903048));
#2793=CARTESIAN_POINT('',(28.0628515535919,0.,-8.54333666903048));
#2794=CARTESIAN_POINT('Ctrl Pts',(48.7532306583709,0.,-7.95408926393383));
#2795=CARTESIAN_POINT('Ctrl Pts',(36.6068452277914,0.,-11.3406614728137));
#2796=CARTESIAN_POINT('Ctrl Pts',(39.4535021242481,0.,-4.7454968822424));
#2797=CARTESIAN_POINT('Ctrl Pts',(31.9355686583357,0.,-5.55619061474896));
#2798=CARTESIAN_POINT('Ctrl Pts',(28.7242328419571,0.,-5.63921626360694));
#2799=CARTESIAN_POINT('Ctrl Pts',(28.0628515535919,0.,-8.54333666903048));
#2800=CARTESIAN_POINT('',(28.0628515535919,1.5,-8.54333666903048));
#2801=CARTESIAN_POINT('',(28.0628515535919,1.5,-8.54333666903048));
#2802=CARTESIAN_POINT('Ctrl Pts',(48.7532306583709,1.5,-7.95408926393383));
#2803=CARTESIAN_POINT('Ctrl Pts',(36.6068452277914,1.5,-11.3406614728137));
#2804=CARTESIAN_POINT('Ctrl Pts',(39.4535021242481,1.5,-4.7454968822424));
#2805=CARTESIAN_POINT('Ctrl Pts',(31.9355686583357,1.5,-5.55619061474896));
#2806=CARTESIAN_POINT('Ctrl Pts',(28.7242328419571,1.5,-5.63921626360694));
#2807=CARTESIAN_POINT('Ctrl Pts',(28.0628515535919,1.5,-8.54333666903048));
#2808=CARTESIAN_POINT('Ctrl Pts',(28.0628515535919,1.5,-8.54333666903048));
#2809=CARTESIAN_POINT('Ctrl Pts',(28.0628515535919,-0.660000000473272,-8.54333666903048));
#2810=CARTESIAN_POINT('Ctrl Pts',(25.2439018750637,1.5,-8.53533145112329));
#2811=CARTESIAN_POINT('Ctrl Pts',(25.2439018750637,-0.660000000473272,-8.53533145112329));
#2812=CARTESIAN_POINT('Ctrl Pts',(10.2818042790062,1.5,-8.66732731527297));
#2813=CARTESIAN_POINT('Ctrl Pts',(10.2818042790062,-0.660000000473272,-8.66732731527297));
#2814=CARTESIAN_POINT('Ctrl Pts',(-10.8727124848744,1.5,-9.29910974996734));
#2815=CARTESIAN_POINT('Ctrl Pts',(-10.8727124848744,-0.660000000473272,
-9.29910974996734));
#2816=CARTESIAN_POINT('Ctrl Pts',(-35.4046976733781,1.5,-5.36519475551457));
#2817=CARTESIAN_POINT('Ctrl Pts',(-35.4046976733781,-0.660000000473272,
-5.36519475551457));
#2818=CARTESIAN_POINT('Ctrl Pts',(-46.8925527716544,1.5,0.201186051515265));
#2819=CARTESIAN_POINT('Ctrl Pts',(-46.8925527716544,-0.660000000473272,
0.201186051515265));
#2820=CARTESIAN_POINT('Ctrl Pts',(-51.680694477123,1.5,4.4617348855033));
#2821=CARTESIAN_POINT('Ctrl Pts',(-51.680694477123,-0.660000000473272,4.4617348855033));
#2822=CARTESIAN_POINT('',(-51.6806944520712,7.01907565403559E-9,4.4617348606735));
#2823=CARTESIAN_POINT('Ctrl Pts',(28.0628515535919,0.,-8.54333666903048));
#2824=CARTESIAN_POINT('Ctrl Pts',(25.2439018750637,0.,-8.53533145112329));
#2825=CARTESIAN_POINT('Ctrl Pts',(10.2818042790062,0.,-8.66732731527297));
#2826=CARTESIAN_POINT('Ctrl Pts',(-10.8727124848744,0.,-9.29910974996734));
#2827=CARTESIAN_POINT('Ctrl Pts',(-35.4046976617966,0.,-5.36519475737177));
#2828=CARTESIAN_POINT('Ctrl Pts',(-46.892552750304,0.,0.201186041170038));
#2829=CARTESIAN_POINT('Ctrl Pts',(-51.6806944508158,0.,4.46173486209483));
#2830=CARTESIAN_POINT('',(-50.5272419105718,1.5,3.47897350344959));
#2831=CARTESIAN_POINT('Ctrl Pts',(-51.6806944612578,2.10963722047097E-8,
4.46173487138622));
#2832=CARTESIAN_POINT('Ctrl Pts',(-51.433849902908,0.328235390347009,4.24208947267881));
#2833=CARTESIAN_POINT('Ctrl Pts',(-51.1892976355325,0.648631772383023,4.03075620524778));
#2834=CARTESIAN_POINT('Ctrl Pts',(-50.9474658918659,0.961189167121584,3.82721318363075));
#2835=CARTESIAN_POINT('Ctrl Pts',(-50.806440496671,1.14345858074691,3.70851604888949));
#2836=CARTESIAN_POINT('Ctrl Pts',(-50.666339525841,1.32306219171186,3.59246881728103));
#2837=CARTESIAN_POINT('Ctrl Pts',(-50.5272419105718,1.5,3.47897350344958));
#2838=CARTESIAN_POINT('Ctrl Pts',(28.0628515535919,1.5,-8.54333666903048));
#2839=CARTESIAN_POINT('Ctrl Pts',(25.2439018750637,1.5,-8.53533145112329));
#2840=CARTESIAN_POINT('Ctrl Pts',(10.2818042790062,1.5,-8.66732731527297));
#2841=CARTESIAN_POINT('Ctrl Pts',(-10.8727124848744,1.5,-9.29910974996734));
#2842=CARTESIAN_POINT('Ctrl Pts',(-34.9052983608708,1.5,-5.4452777340667));
#2843=CARTESIAN_POINT('Ctrl Pts',(-45.9703553177735,1.5,-0.239172727476468));
#2844=CARTESIAN_POINT('Ctrl Pts',(-50.5272419105718,1.5,3.47897350344959));
#2845=CARTESIAN_POINT('Origin',(1.90003279625137,1.5,8.11589060443533));
#2846=CARTESIAN_POINT('',(21.5644964975589,1.49999999962684,4.16303199048503));
#2847=CARTESIAN_POINT('Ctrl Pts',(-50.5272419105718,1.50000000000001,3.4789735034496));
#2848=CARTESIAN_POINT('Ctrl Pts',(-50.5089293710935,1.50000000000002,3.494919364608));
#2849=CARTESIAN_POINT('Ctrl Pts',(-50.490585009579,1.50000000000002,3.51082303253495));
#2850=CARTESIAN_POINT('Ctrl Pts',(-50.472208669657,1.50000000000003,3.5266846817746));
#2851=CARTESIAN_POINT('Ctrl Pts',(-50.4314411765197,1.50000000000004,3.56187339069447));
#2852=CARTESIAN_POINT('Ctrl Pts',(-50.3905163002735,1.50000000000005,3.59685530223419));
#2853=CARTESIAN_POINT('Ctrl Pts',(-50.3494323020579,1.50000000000006,3.63163228677637));
#2854=CARTESIAN_POINT('Ctrl Pts',(-50.2671881545655,1.50000000000008,3.70125071658485));
#2855=CARTESIAN_POINT('Ctrl Pts',(-50.1842968962082,1.5000000000001,3.77005537571968));
#2856=CARTESIAN_POINT('Ctrl Pts',(-50.1007725161627,1.50000000000012,3.83803845959699));
#2857=CARTESIAN_POINT('Ctrl Pts',(-50.0171711659525,1.50000000000013,3.90608419187893));
#2858=CARTESIAN_POINT('Ctrl Pts',(-49.9328424659519,1.50000000000015,3.97337933108099));
#2859=CARTESIAN_POINT('Ctrl Pts',(-49.8480096700854,1.50000000000016,4.03975178559884));
#2860=CARTESIAN_POINT('Ctrl Pts',(-49.763130854313,1.50000000000017,4.10616024569771));
#2861=CARTESIAN_POINT('Ctrl Pts',(-49.6778155128328,1.50000000000018,4.17159851421962));
#2862=CARTESIAN_POINT('Ctrl Pts',(-49.5920096605213,1.50000000000018,4.23611727603634));
#2863=CARTESIAN_POINT('Ctrl Pts',(-49.3831630067192,1.5000000000002,4.3931523400779));
#2864=CARTESIAN_POINT('Ctrl Pts',(-49.1715354999119,1.50000000000021,4.54469690390822));
#2865=CARTESIAN_POINT('Ctrl Pts',(-48.9569720150866,1.50000000000021,4.69110256404027));
#2866=CARTESIAN_POINT('Ctrl Pts',(-48.8191090810188,1.5000000000002,4.78517222312685));
#2867=CARTESIAN_POINT('Ctrl Pts',(-48.6800335406078,1.5000000000002,4.87711933779923));
#2868=CARTESIAN_POINT('Ctrl Pts',(-48.5396990336734,1.5000000000002,4.96702716533848));
#2869=CARTESIAN_POINT('Ctrl Pts',(-48.3121370230267,1.50000000000019,5.11281886300889));
#2870=CARTESIAN_POINT('Ctrl Pts',(-48.0812724142786,1.50000000000017,5.25325158941465));
#2871=CARTESIAN_POINT('Ctrl Pts',(-47.8469042857071,1.50000000000016,5.38865160350329));
#2872=CARTESIAN_POINT('Ctrl Pts',(-47.7137848477506,1.50000000000015,5.46555785302046));
#2873=CARTESIAN_POINT('Ctrl Pts',(-47.5795346580899,1.50000000000015,5.54083958227443));
#2874=CARTESIAN_POINT('Ctrl Pts',(-47.4441134822786,1.50000000000014,5.61454999218334));
#2875=CARTESIAN_POINT('Ctrl Pts',(-47.259034597612,1.50000000000013,5.71528933647368));
#2876=CARTESIAN_POINT('Ctrl Pts',(-47.0717688974148,1.50000000000013,5.81309447963658));
#2877=CARTESIAN_POINT('Ctrl Pts',(-46.8822088597417,1.50000000000013,5.90809195718259));
#2878=CARTESIAN_POINT('Ctrl Pts',(-46.8348188503235,1.50000000000013,5.9318413265691));
#2879=CARTESIAN_POINT('Ctrl Pts',(-46.7872854082889,1.50000000000013,5.95541514647583));
#2880=CARTESIAN_POINT('Ctrl Pts',(-46.7396067820982,1.50000000000013,5.97881525622759));
#2881=CARTESIAN_POINT('Ctrl Pts',(-46.7199618861861,1.50000000000013,5.98845674041312));
#2882=CARTESIAN_POINT('Ctrl Pts',(-46.7002923425438,1.50000000000013,5.99806873380921));
#2883=CARTESIAN_POINT('Ctrl Pts',(-46.6805980273042,1.50000000000013,6.00765136247301));
#2884=CARTESIAN_POINT('Ctrl Pts',(-46.6648305246838,1.50000000000013,6.01532332876016));
#2885=CARTESIAN_POINT('Ctrl Pts',(-46.6490504808134,1.50000000000013,6.02297484102085));
#2886=CARTESIAN_POINT('Ctrl Pts',(-46.6332652127553,1.50000000000013,6.03060245491615));
#2887=CARTESIAN_POINT('Ctrl Pts',(-46.5252097159921,1.50000000000013,6.08281605088054));
#2888=CARTESIAN_POINT('Ctrl Pts',(-46.4168069941106,1.50000000000013,6.13395988895373));
#2889=CARTESIAN_POINT('Ctrl Pts',(-46.3080494255617,1.50000000000013,6.18407421621587));
#2890=CARTESIAN_POINT('Ctrl Pts',(-46.0636310833144,1.50000000000013,6.29669958064508));
#2891=CARTESIAN_POINT('Ctrl Pts',(-45.8174223520571,1.50000000000013,6.40412874272659));
#2892=CARTESIAN_POINT('Ctrl Pts',(-45.5693210884823,1.50000000000013,6.50678841117317));
#2893=CARTESIAN_POINT('Ctrl Pts',(-45.4249966183997,1.50000000000013,6.56650718097678));
#2894=CARTESIAN_POINT('Ctrl Pts',(-45.2800312517206,1.50000000000013,6.62461106801737));
#2895=CARTESIAN_POINT('Ctrl Pts',(-45.1344011822198,1.50000000000013,6.68117694095506));
#2896=CARTESIAN_POINT('Ctrl Pts',(-44.9356631218391,1.50000000000012,6.75837110772237));
#2897=CARTESIAN_POINT('Ctrl Pts',(-44.7356876247125,1.50000000000012,6.83270186595495));
#2898=CARTESIAN_POINT('Ctrl Pts',(-44.5344076135208,1.50000000000012,6.90435191010508));
#2899=CARTESIAN_POINT('Ctrl Pts',(-44.3329812651719,1.50000000000012,6.97605404618287));
#2900=CARTESIAN_POINT('Ctrl Pts',(-44.1303200350267,1.50000000000011,7.04504802588197));
#2901=CARTESIAN_POINT('Ctrl Pts',(-43.926134663197,1.50000000000011,7.11157322203004));
#2902=CARTESIAN_POINT('Ctrl Pts',(-43.7220782177405,1.50000000000011,7.17805641295422));
#2903=CARTESIAN_POINT('Ctrl Pts',(-43.5172432493375,1.50000000000011,7.24182553985641));
#2904=CARTESIAN_POINT('Ctrl Pts',(-43.3120488965543,1.50000000000011,7.30294907653924));
#2905=CARTESIAN_POINT('Ctrl Pts',(-43.1072612505232,1.50000000000011,7.36395146293336));
#2906=CARTESIAN_POINT('Ctrl Pts',(-42.9019014984407,1.5000000000001,7.42238837429228));
#2907=CARTESIAN_POINT('Ctrl Pts',(-42.6959208043633,1.5000000000001,7.47845450070467));
#2908=CARTESIAN_POINT('Ctrl Pts',(-42.6042549864767,1.5000000000001,7.50340512705508));
#2909=CARTESIAN_POINT('Ctrl Pts',(-42.5124595070062,1.50000000000011,7.5278886704349));
#2910=CARTESIAN_POINT('Ctrl Pts',(-42.4205241992551,1.50000000000011,7.55192185945589));
#2911=CARTESIAN_POINT('Ctrl Pts',(-42.4032863290518,1.50000000000011,7.55642808239732));
#2912=CARTESIAN_POINT('Ctrl Pts',(-42.3860435428921,1.50000000000011,7.56091847155628));
#2913=CARTESIAN_POINT('Ctrl Pts',(-42.3687957735994,1.50000000000011,7.56539313583066));
#2914=CARTESIAN_POINT('Ctrl Pts',(-42.3601728119863,1.50000000000011,7.56763022850131));
#2915=CARTESIAN_POINT('Ctrl Pts',(-42.3515486048558,1.50000000000011,7.56986339078578));
#2916=CARTESIAN_POINT('Ctrl Pts',(-42.3429231438093,1.50000000000011,7.57209263625319));
#2917=CARTESIAN_POINT('Ctrl Pts',(-42.3387712046192,1.50000000000011,7.5731657025589));
#2918=CARTESIAN_POINT('Ctrl Pts',(-42.3346189748892,1.50000000000011,7.57423786131412));
#2919=CARTESIAN_POINT('Ctrl Pts',(-42.3304664536822,1.50000000000011,7.57530911403014));
#2920=CARTESIAN_POINT('Ctrl Pts',(-42.3268345793521,1.50000000000011,7.57624605210858));
#2921=CARTESIAN_POINT('Ctrl Pts',(-42.3231990849173,1.50000000000011,7.57718317460447));
#2922=CARTESIAN_POINT('Ctrl Pts',(-42.3195518619974,1.50000000000011,7.57812256321697));
#2923=CARTESIAN_POINT('Ctrl Pts',(-42.206229235501,1.50000000000011,7.60731024579269));
#2924=CARTESIAN_POINT('Ctrl Pts',(-42.0838991388229,1.50000000000011,7.63809273955698));
#2925=CARTESIAN_POINT('Ctrl Pts',(-41.9519336281348,1.50000000000011,7.67029075065104));
#2926=CARTESIAN_POINT('Ctrl Pts',(-41.8145918531791,1.50000000000011,7.70380050612157));
#2927=CARTESIAN_POINT('Ctrl Pts',(-41.6668135148127,1.50000000000011,7.73884328952492));
#2928=CARTESIAN_POINT('Ctrl Pts',(-41.5078848858298,1.50000000000011,7.77516083651302));
#2929=CARTESIAN_POINT('Ctrl Pts',(-41.4914728560587,1.50000000000011,7.77891122853614));
#2930=CARTESIAN_POINT('Ctrl Pts',(-41.4749419152315,1.50000000000011,7.78267516942519));
#2931=CARTESIAN_POINT('Ctrl Pts',(-41.4582912745849,1.50000000000011,7.78645234462284));
#2932=CARTESIAN_POINT('Ctrl Pts',(-41.2880437092141,1.50000000000011,7.82507277341156));
#2933=CARTESIAN_POINT('Ctrl Pts',(-41.105280703604,1.50000000000011,7.86508066099839));
#2934=CARTESIAN_POINT('Ctrl Pts',(-40.9091507676617,1.50000000000011,7.90609878628782));
#2935=CARTESIAN_POINT('Ctrl Pts',(-40.6940198379218,1.50000000000011,7.95109073199615));
#2936=CARTESIAN_POINT('Ctrl Pts',(-40.4628063102105,1.50000000000011,7.997296187756));
#2937=CARTESIAN_POINT('Ctrl Pts',(-40.21437984959,1.50000000000011,8.0441643485791));
#2938=CARTESIAN_POINT('Ctrl Pts',(-39.8881230599814,1.50000000000011,8.105715987027));
#2939=CARTESIAN_POINT('Ctrl Pts',(-39.5321785961021,1.50000000000011,8.16841177106708));
#2940=CARTESIAN_POINT('Ctrl Pts',(-39.1439725199136,1.50000000000011,8.23089497229237));
#2941=CARTESIAN_POINT('Ctrl Pts',(-38.9161892647587,1.50000000000011,8.2675575281888));
#2942=CARTESIAN_POINT('Ctrl Pts',(-38.6772986944323,1.50000000000011,8.30414605659786));
#2943=CARTESIAN_POINT('Ctrl Pts',(-38.4267841261925,1.50000000000011,8.34041277840537));
#2944=CARTESIAN_POINT('Ctrl Pts',(-38.1981544821903,1.50000000000011,8.37351124351358));
#2945=CARTESIAN_POINT('Ctrl Pts',(-37.9598429527006,1.50000000000011,8.40634072421756));
#2946=CARTESIAN_POINT('Ctrl Pts',(-37.7114615095564,1.50000000000011,8.43875071588523));
#2947=CARTESIAN_POINT('Ctrl Pts',(-37.4786681910349,1.50000000000011,8.46912669493609));
#2948=CARTESIAN_POINT('Ctrl Pts',(-37.2370280971275,1.50000000000011,8.4991249687636));
#2949=CARTESIAN_POINT('Ctrl Pts',(-36.9862244620814,1.50000000000011,8.52864320020706));
#2950=CARTESIAN_POINT('Ctrl Pts',(-36.8132513602342,1.50000000000011,8.54900119881773));
#2951=CARTESIAN_POINT('Ctrl Pts',(-36.6359196923416,1.50000000000011,8.56913160302865));
#2952=CARTESIAN_POINT('Ctrl Pts',(-36.454127373203,1.50000000000011,8.58901547789096));
#2953=CARTESIAN_POINT('Ctrl Pts',(-36.2135217073827,1.50000000000011,8.61533217252913));
#2954=CARTESIAN_POINT('Ctrl Pts',(-35.9651025463024,1.50000000000011,8.6412189721965));
#2955=CARTESIAN_POINT('Ctrl Pts',(-35.7086359890007,1.50000000000011,8.66665419066998));
#2956=CARTESIAN_POINT('Ctrl Pts',(-35.540534914934,1.50000000000011,8.68332571146979));
#2957=CARTESIAN_POINT('Ctrl Pts',(-35.3689766642997,1.50000000000011,8.69980407477762));
#2958=CARTESIAN_POINT('Ctrl Pts',(-35.1938969052879,1.5000000000001,8.71609544289402));
#2959=CARTESIAN_POINT('Ctrl Pts',(-34.7919055046781,1.5000000000001,8.7535011939867));
#2960=CARTESIAN_POINT('Ctrl Pts',(-34.3713714780771,1.5000000000001,8.79009866226096));
#2961=CARTESIAN_POINT('Ctrl Pts',(-33.9314440825312,1.5000000000001,8.82538571608246));
#2962=CARTESIAN_POINT('Ctrl Pts',(-33.7268155351118,1.5000000000001,8.8417991939411));
#2963=CARTESIAN_POINT('Ctrl Pts',(-33.5179894076552,1.5000000000001,8.85791559409581));
#2964=CARTESIAN_POINT('Ctrl Pts',(-33.304877686204,1.5000000000001,8.87366518630366));
#2965=CARTESIAN_POINT('Ctrl Pts',(-33.2920726363165,1.5000000000001,8.87461151770466));
#2966=CARTESIAN_POINT('Ctrl Pts',(-33.2792521138151,1.5000000000001,8.87555652343868));
#2967=CARTESIAN_POINT('Ctrl Pts',(-33.266416099541,1.5000000000001,8.87650018785329));
#2968=CARTESIAN_POINT('Ctrl Pts',(-33.257215426996,1.5000000000001,8.87717659308982));
#2969=CARTESIAN_POINT('Ctrl Pts',(-33.2480165202098,1.5000000000001,8.87785159417242));
#2970=CARTESIAN_POINT('Ctrl Pts',(-33.238819841101,1.5000000000001,8.87852515918472));
#2971=CARTESIAN_POINT('Ctrl Pts',(-33.0473126301575,1.5000000000001,8.89255115219479));
#2972=CARTESIAN_POINT('Ctrl Pts',(-32.856704989813,1.5000000000001,8.90595933266772));
#2973=CARTESIAN_POINT('Ctrl Pts',(-32.6670039177075,1.50000000000009,8.91876754736317));
#2974=CARTESIAN_POINT('Ctrl Pts',(-31.8030452793489,1.50000000000009,8.97710020518771));
#2975=CARTESIAN_POINT('Ctrl Pts',(-30.9578608360811,1.50000000000009,9.02294794423588));
#2976=CARTESIAN_POINT('Ctrl Pts',(-30.1321621754745,1.50000000000008,9.05781079611547));
#2977=CARTESIAN_POINT('Ctrl Pts',(-29.5578848243791,1.50000000000008,9.08205807564277));
#2978=CARTESIAN_POINT('Ctrl Pts',(-28.9928890954127,1.50000000000008,9.10099165420077));
#2979=CARTESIAN_POINT('Ctrl Pts',(-28.4376302401943,1.50000000000007,9.11509773780446));
#2980=CARTESIAN_POINT('Ctrl Pts',(-28.1523110222181,1.50000000000007,9.1223461350244));
#2981=CARTESIAN_POINT('Ctrl Pts',(-27.8695618760832,1.50000000000007,9.12831980439727));
#2982=CARTESIAN_POINT('Ctrl Pts',(-27.5894392714,1.50000000000007,9.13308420054702));
#2983=CARTESIAN_POINT('Ctrl Pts',(-26.9277478962211,1.50000000000006,9.14433841490715));
#2984=CARTESIAN_POINT('Ctrl Pts',(-26.281454611936,1.50000000000006,9.14884113583659));
#2985=CARTESIAN_POINT('Ctrl Pts',(-25.6506510642923,1.50000000000006,9.14749549738845));
#2986=CARTESIAN_POINT('Ctrl Pts',(-25.4470002765794,1.50000000000005,9.14706106684195));
#2987=CARTESIAN_POINT('Ctrl Pts',(-25.244964291622,1.50000000000005,9.14601684953584));
#2988=CARTESIAN_POINT('Ctrl Pts',(-25.0445471446942,1.50000000000005,9.14439258279129));
#2989=CARTESIAN_POINT('Ctrl Pts',(-24.3270447678852,1.50000000000005,9.1385776349804));
#2990=CARTESIAN_POINT('Ctrl Pts',(-23.6303730883905,1.50000000000004,9.12533114326984));
#2991=CARTESIAN_POINT('Ctrl Pts',(-22.9549224301413,1.50000000000004,9.10597228944781));
#2992=CARTESIAN_POINT('Ctrl Pts',(-22.8025170686509,1.50000000000004,9.10160425296912));
#2993=CARTESIAN_POINT('Ctrl Pts',(-22.651192098821,1.50000000000004,9.09692481967301));
#2994=CARTESIAN_POINT('Ctrl Pts',(-22.5009520119949,1.50000000000003,9.09194877207359));
#2995=CARTESIAN_POINT('Ctrl Pts',(-21.8779473032801,1.50000000000003,9.07131445835136));
#2996=CARTESIAN_POINT('Ctrl Pts',(-21.2736303287498,1.50000000000003,9.04557907659367));
#2997=CARTESIAN_POINT('Ctrl Pts',(-20.6882518298076,1.50000000000002,9.01577329099357));
#2998=CARTESIAN_POINT('Ctrl Pts',(-20.441683640011,1.50000000000002,9.00321874959145));
#2999=CARTESIAN_POINT('Ctrl Pts',(-20.1984758287443,1.50000000000002,8.98994150190267));
#3000=CARTESIAN_POINT('Ctrl Pts',(-19.9586485146901,1.50000000000002,8.97601616457639));
#3001=CARTESIAN_POINT('Ctrl Pts',(-19.5918929480637,1.50000000000002,8.95472086298948));
#3002=CARTESIAN_POINT('Ctrl Pts',(-19.2331539217403,1.50000000000001,8.93188131021674));
#3003=CARTESIAN_POINT('Ctrl Pts',(-18.8825930785396,1.50000000000001,8.90789764190378));
#3004=CARTESIAN_POINT('Ctrl Pts',(-18.8175713347727,1.50000000000001,8.90344917035916));
#3005=CARTESIAN_POINT('Ctrl Pts',(-18.7528308756026,1.50000000000001,8.89896120970124));
#3006=CARTESIAN_POINT('Ctrl Pts',(-18.6883726443041,1.50000000000001,8.89443613951083));
#3007=CARTESIAN_POINT('Ctrl Pts',(-18.3254612991177,1.50000000000001,8.86895918681165));
#3008=CARTESIAN_POINT('Ctrl Pts',(-17.9714391298583,1.50000000000001,8.84231305930845));
#3009=CARTESIAN_POINT('Ctrl Pts',(-17.6263903838312,1.50000000000001,8.81489638468738));
#3010=CARTESIAN_POINT('Ctrl Pts',(-17.5571089984659,1.50000000000001,8.80939146626143));
#3011=CARTESIAN_POINT('Ctrl Pts',(-17.4881893783597,1.50000000000001,8.80385531451122));
#3012=CARTESIAN_POINT('Ctrl Pts',(-17.4196322012764,1.50000000000001,8.79829090617308));
#3013=CARTESIAN_POINT('Ctrl Pts',(-17.0698855435987,1.5,8.76990389694932));
#3014=CARTESIAN_POINT('Ctrl Pts',(-16.7295567947277,1.5,8.74078650592042));
#3015=CARTESIAN_POINT('Ctrl Pts',(-16.3987215411361,1.5,8.71130261677436));
#3016=CARTESIAN_POINT('Ctrl Pts',(-16.1344697349496,1.5,8.68775261454312));
#3017=CARTESIAN_POINT('Ctrl Pts',(-15.8762747673998,1.5,8.66396767432586));
#3018=CARTESIAN_POINT('Ctrl Pts',(-15.6241773384801,1.5,8.64011005957217));
#3019=CARTESIAN_POINT('Ctrl Pts',(-15.4981286240202,1.5,8.62818125219533));
#3020=CARTESIAN_POINT('Ctrl Pts',(-15.3736043234866,1.5,8.61623396593671));
#3021=CARTESIAN_POINT('Ctrl Pts',(-15.2506096943136,1.5,8.60428668530748));
#3022=CARTESIAN_POINT('Ctrl Pts',(-15.1891123797271,1.5,8.59831304499287));
#3023=CARTESIAN_POINT('Ctrl Pts',(-15.1279974847049,1.5,8.59233938786278));
#3024=CARTESIAN_POINT('Ctrl Pts',(-15.0672656765957,1.5,8.5863679170989));
#3025=CARTESIAN_POINT('Ctrl Pts',(-15.0368997725411,1.5,8.58338218171695));
#3026=CARTESIAN_POINT('Ctrl Pts',(-15.0066296403192,1.5,8.58039699182383));
#3027=CARTESIAN_POINT('Ctrl Pts',(-14.9764553639702,1.5,8.57741261626164));
#3028=CARTESIAN_POINT('Ctrl Pts',(-14.9571460107395,1.5,8.57550283187321));
#3029=CARTESIAN_POINT('Ctrl Pts',(-14.9378759112039,1.5,8.57359338087164));
#3030=CARTESIAN_POINT('Ctrl Pts',(-14.9186450874746,1.5,8.57168433278082));
#3031=CARTESIAN_POINT('Ctrl Pts',(-14.907824351077,1.5,8.57061015590456));
#3032=CARTESIAN_POINT('Ctrl Pts',(-14.8970170168616,1.5,8.56953620375837));
#3033=CARTESIAN_POINT('Ctrl Pts',(-14.8862060042313,1.5,8.56846078627014));
#3034=CARTESIAN_POINT('Ctrl Pts',(-14.1315605865435,1.5,8.49339299129559));
#3035=CARTESIAN_POINT('Ctrl Pts',(-13.3783601642147,1.5,8.41312271947158));
#3036=CARTESIAN_POINT('Ctrl Pts',(-12.6255306242344,1.5,8.3290249277592));
#3037=CARTESIAN_POINT('Ctrl Pts',(-11.6940973381783,1.50000000000001,8.2249755004655));
#3038=CARTESIAN_POINT('Ctrl Pts',(-10.7632320809417,1.50000000000001,8.11506424364423));
#3039=CARTESIAN_POINT('Ctrl Pts',(-9.83090827917461,1.50000000000002,8.00182359519212));
#3040=CARTESIAN_POINT('Ctrl Pts',(-8.99377176042809,1.50000000000002,7.90014445534165));
#3041=CARTESIAN_POINT('Ctrl Pts',(-8.15545622107017,1.50000000000003,7.79578997275644));
#3042=CARTESIAN_POINT('Ctrl Pts',(-7.31449954828799,1.50000000000003,7.69052599994285));
#3043=CARTESIAN_POINT('Ctrl Pts',(-6.59897401816955,1.50000000000004,7.60096245596069));
#3044=CARTESIAN_POINT('Ctrl Pts',(-5.88153659056765,1.50000000000004,7.51073932052197));
#3045=CARTESIAN_POINT('Ctrl Pts',(-5.16128259334547,1.50000000000004,7.4209820220267));
#3046=CARTESIAN_POINT('Ctrl Pts',(-5.03502255358876,1.50000000000004,7.40524762815984));
#3047=CARTESIAN_POINT('Ctrl Pts',(-4.90867594722178,1.50000000000004,7.38952767781894));
#3048=CARTESIAN_POINT('Ctrl Pts',(-4.78223788163677,1.50000000000004,7.37382841185874));
#3049=CARTESIAN_POINT('Ctrl Pts',(-4.56955323079961,1.50000000000004,7.3474202816513));
#3050=CARTESIAN_POINT('Ctrl Pts',(-4.3566091032761,1.50000000000004,7.32107008947461));
#3051=CARTESIAN_POINT('Ctrl Pts',(-4.1433830569508,1.50000000000004,7.29480646014441));
#3052=CARTESIAN_POINT('Ctrl Pts',(-3.98346352220683,1.50000000000004,7.27510873814677));
#3053=CARTESIAN_POINT('Ctrl Pts',(-3.82338540727857,1.50000000000004,7.25545971747252));
#3054=CARTESIAN_POINT('Ctrl Pts',(-3.66313922667493,1.50000000000004,7.23587167633331));
#3055=CARTESIAN_POINT('Ctrl Pts',(-3.62715621894005,1.50000000000004,7.23147321495864));
#3056=CARTESIAN_POINT('Ctrl Pts',(-3.59116473694397,1.50000000000004,7.22707782902003));
#3057=CARTESIAN_POINT('Ctrl Pts',(-3.55516467317788,1.50000000000004,7.22268565882026));
#3058=CARTESIAN_POINT('Ctrl Pts',(-3.54355314240601,1.50000000000004,7.22126899967873));
#3059=CARTESIAN_POINT('Ctrl Pts',(-3.53194448754217,1.50000000000004,7.21985313509436));
#3060=CARTESIAN_POINT('Ctrl Pts',(-3.52034685551296,1.50000000000004,7.21843906205996));
#3061=CARTESIAN_POINT('Ctrl Pts',(-3.11130718235708,1.50000000000004,7.16856578013871));
#3062=CARTESIAN_POINT('Ctrl Pts',(-2.71295083324768,1.50000000000004,7.12055605910502));
#3063=CARTESIAN_POINT('Ctrl Pts',(-2.32483672197188,1.50000000000004,7.07445773148509));
#3064=CARTESIAN_POINT('Ctrl Pts',(-2.30225766518038,1.50000000000004,7.07177589970654));
#3065=CARTESIAN_POINT('Ctrl Pts',(-2.27971327425372,1.50000000000004,7.0691005226414));
#3066=CARTESIAN_POINT('Ctrl Pts',(-2.25720346275927,1.50000000000004,7.06643160452515));
#3067=CARTESIAN_POINT('Ctrl Pts',(-1.80960285994172,1.50000000000004,7.01336099760358));
#3068=CARTESIAN_POINT('Ctrl Pts',(-1.37567372863184,1.50000000000004,6.96285895545701));
#3069=CARTESIAN_POINT('Ctrl Pts',(-0.954738519600669,1.50000000000004,6.9148961501584));
#3070=CARTESIAN_POINT('Ctrl Pts',(-0.533803310569499,1.50000000000004,6.86693334485979));
#3071=CARTESIAN_POINT('Ctrl Pts',(-0.125862135491728,1.50000000000004,6.82150863908376));
#3072=CARTESIAN_POINT('Ctrl Pts',(0.269757237238929,1.50000000000004,6.77853867313061));
#3073=CARTESIAN_POINT('Ctrl Pts',(0.705941810521693,1.50000000000004,6.73116274172998));
#3074=CARTESIAN_POINT('Ctrl Pts',(1.12715344954864,1.50000000000004,6.68682581445775));
#3075=CARTESIAN_POINT('Ctrl Pts',(1.53428028329925,1.50000000000004,6.64528629088636));
#3076=CARTESIAN_POINT('Ctrl Pts',(1.87215098302727,1.50000000000004,6.61081303407316));
#3077=CARTESIAN_POINT('Ctrl Pts',(2.2003275842666,1.50000000000004,6.57833169383247));
#3078=CARTESIAN_POINT('Ctrl Pts',(2.51930177206597,1.50000000000004,6.54754073376113));
#3079=CARTESIAN_POINT('Ctrl Pts',(2.61354920273931,1.50000000000004,6.53844291649037));
#3080=CARTESIAN_POINT('Ctrl Pts',(2.70699327148389,1.50000000000004,6.5294930242348));
#3081=CARTESIAN_POINT('Ctrl Pts',(2.79964674389792,1.50000000000004,6.52068412397982));
#3082=CARTESIAN_POINT('Ctrl Pts',(3.10485723459384,1.50000000000003,6.49166666031369));
#3083=CARTESIAN_POINT('Ctrl Pts',(3.40148201654041,1.50000000000003,6.46410905983882));
#3084=CARTESIAN_POINT('Ctrl Pts',(3.68997607232203,1.50000000000003,6.43774996449062));
#3085=CARTESIAN_POINT('Ctrl Pts',(3.99784226211859,1.50000000000003,6.40962087798535));
#3086=CARTESIAN_POINT('Ctrl Pts',(4.29644914071748,1.50000000000003,6.38285685673465));
#3087=CARTESIAN_POINT('Ctrl Pts',(4.58635565562216,1.50000000000003,6.35720199708492));
#3088=CARTESIAN_POINT('Ctrl Pts',(4.84164454089151,1.50000000000003,6.33461057472978));
#3089=CARTESIAN_POINT('Ctrl Pts',(5.09018694388211,1.50000000000003,6.31288049665803));
#3090=CARTESIAN_POINT('Ctrl Pts',(5.33236776508438,1.50000000000003,6.29187011097832));
#3091=CARTESIAN_POINT('Ctrl Pts',(5.6345644513341,1.50000000000003,6.26565305176728));
#3092=CARTESIAN_POINT('Ctrl Pts',(5.92685513364938,1.50000000000003,6.24054875616991));
#3093=CARTESIAN_POINT('Ctrl Pts',(6.20999223681358,1.50000000000003,6.21632922031447));
#3094=CARTESIAN_POINT('Ctrl Pts',(6.52078059810494,1.50000000000002,6.18974439700579));
#3095=CARTESIAN_POINT('Ctrl Pts',(6.82054022294184,1.50000000000002,6.16422587194136));
#3096=CARTESIAN_POINT('Ctrl Pts',(7.11027273672712,1.50000000000002,6.13953902411822));
#3097=CARTESIAN_POINT('Ctrl Pts',(7.37008754579113,1.50000000000002,6.11740133384052));
#3098=CARTESIAN_POINT('Ctrl Pts',(7.62183926725666,1.50000000000002,6.09593391271264));
#3099=CARTESIAN_POINT('Ctrl Pts',(7.86625360733992,1.50000000000002,6.07500271807589));
#3100=CARTESIAN_POINT('Ctrl Pts',(8.09291279008128,1.50000000000002,6.05559204246434));
#3101=CARTESIAN_POINT('Ctrl Pts',(8.31326296260427,1.50000000000002,6.03664426550279));
#3102=CARTESIAN_POINT('Ctrl Pts',(8.52788366706357,1.50000000000002,6.01806828389815));
#3103=CARTESIAN_POINT('Ctrl Pts',(8.68884919540805,1.50000000000002,6.00413629769468));
#3104=CARTESIAN_POINT('Ctrl Pts',(8.84659194283416,1.50000000000002,5.99041384636439));
#3105=CARTESIAN_POINT('Ctrl Pts',(9.00135696938046,1.50000000000002,5.9768675024729));
#3106=CARTESIAN_POINT('Ctrl Pts',(9.01581102489525,1.50000000000002,5.97560236130374));
#3107=CARTESIAN_POINT('Ctrl Pts',(9.03023910795808,1.50000000000002,5.97433875874388));
#3108=CARTESIAN_POINT('Ctrl Pts',(9.04464141836935,1.50000000000002,5.97307666907199));
#3109=CARTESIAN_POINT('Ctrl Pts',(9.05358082167618,1.50000000000002,5.97229329971913));
#3110=CARTESIAN_POINT('Ctrl Pts',(9.06250938704645,1.50000000000002,5.97151059322107));
#3111=CARTESIAN_POINT('Ctrl Pts',(9.07144369583731,1.50000000000002,5.97072709265066));
#3112=CARTESIAN_POINT('Ctrl Pts',(9.51048454911024,1.50000000000002,5.93222509243753));
#3113=CARTESIAN_POINT('Ctrl Pts',(9.95403537666102,1.50000000000002,5.8926258316374));
#3114=CARTESIAN_POINT('Ctrl Pts',(10.3995073164968,1.50000000000002,5.85165205131927));
#3115=CARTESIAN_POINT('Ctrl Pts',(10.8207555645272,1.50000000000002,5.81290632654801));
#3116=CARTESIAN_POINT('Ctrl Pts',(11.2437548001683,1.50000000000002,5.77293047513436));
#3117=CARTESIAN_POINT('Ctrl Pts',(11.6662637360807,1.50000000000002,5.73147701131878));
#3118=CARTESIAN_POINT('Ctrl Pts',(12.0374006682032,1.50000000000002,5.69506379001463));
#3119=CARTESIAN_POINT('Ctrl Pts',(12.4081589691877,1.50000000000001,5.65750947828726));
#3120=CARTESIAN_POINT('Ctrl Pts',(12.7770243679439,1.50000000000001,5.61868654953851));
#3121=CARTESIAN_POINT('Ctrl Pts',(12.8280819508003,1.50000000000001,5.61331276032435));
#3122=CARTESIAN_POINT('Ctrl Pts',(12.8791032787792,1.50000000000001,5.60791474655984));
#3123=CARTESIAN_POINT('Ctrl Pts',(12.9300843489308,1.50000000000001,5.60249225367133));
#3124=CARTESIAN_POINT('Ctrl Pts',(13.2595479279469,1.50000000000001,5.56744956216012));
#3125=CARTESIAN_POINT('Ctrl Pts',(13.5873394667212,1.50000000000001,5.53138422159486));
#3126=CARTESIAN_POINT('Ctrl Pts',(13.9123956890807,1.50000000000001,5.49422080575756));
#3127=CARTESIAN_POINT('Ctrl Pts',(14.2186795743761,1.50000000000001,5.45920361608227));
#3128=CARTESIAN_POINT('Ctrl Pts',(14.5225349237245,1.50000000000001,5.42321129865508));
#3129=CARTESIAN_POINT('Ctrl Pts',(14.8230783860206,1.50000000000001,5.38622616438368));
#3130=CARTESIAN_POINT('Ctrl Pts',(15.035316648525,1.50000000000001,5.36010794315775));
#3131=CARTESIAN_POINT('Ctrl Pts',(15.2459034227506,1.50000000000001,5.33349553417475));
#3132=CARTESIAN_POINT('Ctrl Pts',(15.454529747749,1.50000000000001,5.30639838000327));
#3133=CARTESIAN_POINT('Ctrl Pts',(15.7314585932908,1.50000000000001,5.27042984332779));
#3134=CARTESIAN_POINT('Ctrl Pts',(16.0049330589367,1.50000000000001,5.23360279460352));
#3135=CARTESIAN_POINT('Ctrl Pts',(16.2742336283039,1.5,5.19595898559869));
#3136=CARTESIAN_POINT('Ctrl Pts',(16.4219131180616,1.5,5.17531581161865));
#3137=CARTESIAN_POINT('Ctrl Pts',(16.5683375408946,1.5,5.15442789297188));
#3138=CARTESIAN_POINT('Ctrl Pts',(16.7133891339298,1.5,5.13330876447839));
#3139=CARTESIAN_POINT('Ctrl Pts',(16.9684975087711,1.5,5.09616565949551));
#3140=CARTESIAN_POINT('Ctrl Pts',(17.2193592251396,1.5,5.05830547382683));
#3141=CARTESIAN_POINT('Ctrl Pts',(17.4653369451222,1.5,5.01982643614904));
#3142=CARTESIAN_POINT('Ctrl Pts',(17.635772215158,1.5,4.9931647320817));
#3143=CARTESIAN_POINT('Ctrl Pts',(17.8038628427899,1.5,4.96620697017877));
#3144=CARTESIAN_POINT('Ctrl Pts',(17.9693987744903,1.5,4.93900041044443));
#3145=CARTESIAN_POINT('Ctrl Pts',(18.1827156839134,1.5,4.90394083649605));
#3146=CARTESIAN_POINT('Ctrl Pts',(18.3917899704582,1.5,4.86846598332765));
#3147=CARTESIAN_POINT('Ctrl Pts',(18.5961751592073,1.5,4.83269950369486));
#3148=CARTESIAN_POINT('Ctrl Pts',(18.7017980573384,1.5,4.81421597630288));
#3149=CARTESIAN_POINT('Ctrl Pts',(18.806168729909,1.5,4.7956550811478));
#3150=CARTESIAN_POINT('Ctrl Pts',(18.9092259812001,1.5,4.77703704590836));
#3151=CARTESIAN_POINT('Ctrl Pts',(19.0149000522275,1.5,4.7579462633226));
#3152=CARTESIAN_POINT('Ctrl Pts',(19.1191939813236,1.5,4.73879804741868));
#3153=CARTESIAN_POINT('Ctrl Pts',(19.2220396298678,1.5,4.71960863557561));
#3154=CARTESIAN_POINT('Ctrl Pts',(19.3277806393804,1.5,4.69987899403062));
#3155=CARTESIAN_POINT('Ctrl Pts',(19.4319522489605,1.5,4.68014548934906));
#3156=CARTESIAN_POINT('Ctrl Pts',(19.5344534591269,1.5,4.66032590026468));
#3157=CARTESIAN_POINT('Ctrl Pts',(19.6401702303914,1.5,4.63988455169533));
#3158=CARTESIAN_POINT('Ctrl Pts',(19.7441057609561,1.5,4.61933682528627));
#3159=CARTESIAN_POINT('Ctrl Pts',(19.8461483400865,1.5,4.5985899959703));
#3160=CARTESIAN_POINT('Ctrl Pts',(19.9603425121877,1.5,4.57537256048748));
#3161=CARTESIAN_POINT('Ctrl Pts',(20.0721640111897,1.5,4.55189882105127));
#3162=CARTESIAN_POINT('Ctrl Pts',(20.1814687083029,1.5,4.52808124461801));
#3163=CARTESIAN_POINT('Ctrl Pts',(20.2784032176319,1.5,4.50695914148847));
#3164=CARTESIAN_POINT('Ctrl Pts',(20.3733585787686,1.5,4.48556739870102));
#3165=CARTESIAN_POINT('Ctrl Pts',(20.466243911377,1.5,4.46387787110044));
#3166=CARTESIAN_POINT('Ctrl Pts',(20.5763630626326,1.5,4.43816409796275));
#3167=CARTESIAN_POINT('Ctrl Pts',(20.6835711433518,1.5,4.41202618656764));
#3168=CARTESIAN_POINT('Ctrl Pts',(20.7877374720262,1.5,4.38548804258589));
#3169=CARTESIAN_POINT('Ctrl Pts',(20.8880371211572,1.5,4.3599350009857));
#3170=CARTESIAN_POINT('Ctrl Pts',(20.9855167974935,1.5,4.33401139842294));
#3171=CARTESIAN_POINT('Ctrl Pts',(21.0800726838929,1.5,4.30778240560577));
#3172=CARTESIAN_POINT('Ctrl Pts',(21.1899754169482,1.5,4.27729632900427));
#3173=CARTESIAN_POINT('Ctrl Pts',(21.2959271796799,1.5,4.24639403035665));
#3174=CARTESIAN_POINT('Ctrl Pts',(21.3977943899266,1.5,4.21527827297281));
#3175=CARTESIAN_POINT('Ctrl Pts',(21.4546405350168,1.5,4.19791438468579));
#3176=CARTESIAN_POINT('Ctrl Pts',(21.5102149898772,1.5,4.1804849859871));
#3177=CARTESIAN_POINT('Ctrl Pts',(21.5644964972823,1.5,4.16303198962476));
#3178=CARTESIAN_POINT('',(21.3356435067856,1.5,3.73655812712738));
#3179=CARTESIAN_POINT('',(22.5271211105952,1.5,5.95690952216869));
#3180=CARTESIAN_POINT('',(21.3356435067856,1.5,3.73655812712738));
#3181=CARTESIAN_POINT('Origin',(1.90003279625137,0.,8.11589060443533));
#3182=CARTESIAN_POINT('',(21.3356435067856,0.,3.73655812712738));
#3183=CARTESIAN_POINT('',(21.3356435067856,0.,3.73655812712738));
#3184=CARTESIAN_POINT('',(22.284188719917,-3.50719883690508E-10,5.50419830755606));
#3185=CARTESIAN_POINT('',(22.5271211105952,0.,5.95690952216869));
#3186=CARTESIAN_POINT('Ctrl Pts',(-51.6806944441105,-1.50990331349021E-14,
4.46173484851326));
#3187=CARTESIAN_POINT('Ctrl Pts',(-51.6763944115022,5.87692512758708E-13,
4.46557237996829));
#3188=CARTESIAN_POINT('Ctrl Pts',(-51.6717236003112,-1.02756276505808E-14,
4.46973835626723));
#3189=CARTESIAN_POINT('Ctrl Pts',(-51.6618445772489,-1.26565424807279E-14,
4.47853832467601));
#3190=CARTESIAN_POINT('Ctrl Pts',(-51.6562942458247,-1.36557432028894E-14,
4.48347711152442));
#3191=CARTESIAN_POINT('Ctrl Pts',(-51.6399305987615,-1.54321000422896E-14,
4.49801845622271));
#3192=CARTESIAN_POINT('Ctrl Pts',(-51.6289127938884,-1.63757896132209E-14,
4.50778632959587));
#3193=CARTESIAN_POINT('Ctrl Pts',(-51.6069503571003,-1.63757896132212E-14,
4.52720927807316));
#3194=CARTESIAN_POINT('Ctrl Pts',(-51.5959572964355,-1.54321000422898E-14,
4.53690769597779));
#3195=CARTESIAN_POINT('Ctrl Pts',(-51.5629426093583,-9.71445146546972E-15,
4.56596373819379));
#3196=CARTESIAN_POINT('Ctrl Pts',(-51.5188283460193,-1.97064586869581E-14,
4.60460056353571));
#3197=CARTESIAN_POINT('Ctrl Pts',(-51.4745249624866,-1.48214773787458E-14,
4.64302781421577));
#3198=CARTESIAN_POINT('Ctrl Pts',(-51.4079282366868,-5.60662627435695E-15,
4.70051118190272));
#3199=CARTESIAN_POINT('Ctrl Pts',(-51.3633415497112,-1.40998324127395E-14,
4.73862341351609));
#3200=CARTESIAN_POINT('Ctrl Pts',(-51.229016501315,-9.99200722162641E-15,
4.85232753950401));
#3201=CARTESIAN_POINT('Ctrl Pts',(-51.13870277151,-1.55431223447521E-14,
4.92729489364781));
#3202=CARTESIAN_POINT('Ctrl Pts',(-50.956619740663,-1.47104550762833E-14,
5.0754979207133));
#3203=CARTESIAN_POINT('Ctrl Pts',(-50.8647490823044,-1.55431223447522E-14,
5.14881255305296));
#3204=CARTESIAN_POINT('Ctrl Pts',(-50.6798803771769,-1.47104550762833E-14,
5.29345224746616));
#3205=CARTESIAN_POINT('Ctrl Pts',(-50.5869566911128,-1.51545442861334E-14,
5.36472658268942));
#3206=CARTESIAN_POINT('Ctrl Pts',(-50.1197141929288,-9.82547376793259E-15,
5.71605324160813));
#3207=CARTESIAN_POINT('Ctrl Pts',(-49.7378902077951,-1.52655665885959E-14,
5.98082374985693));
#3208=CARTESIAN_POINT('Ctrl Pts',(-48.9598663397128,-1.52655665885959E-14,
6.47927805260146));
#3209=CARTESIAN_POINT('Ctrl Pts',(-48.5636892956867,-1.52655665885959E-14,
6.71296610783997));
#3210=CARTESIAN_POINT('Ctrl Pts',(-47.7587593461934,-1.52655665885959E-14,
7.15109273394721));
#3211=CARTESIAN_POINT('Ctrl Pts',(-47.3500098510032,-1.47104550762833E-14,
7.3555359494196));
#3212=CARTESIAN_POINT('Ctrl Pts',(-46.5215810175673,-1.55431223447522E-14,
7.73726655172034));
#3213=CARTESIAN_POINT('Ctrl Pts',(-46.1019027012514,-1.46549439250521E-14,
7.91455864407753));
#3214=CARTESIAN_POINT('Ctrl Pts',(-45.4653032959013,-1.32116539930394E-14,
8.16182742932691));
#3215=CARTESIAN_POINT('Ctrl Pts',(-45.251921935563,-1.07136521876328E-14,
8.24114014723876));
#3216=CARTESIAN_POINT('Ctrl Pts',(-44.8229670778109,-1.23234755733392E-14,
8.39383604775355));
#3217=CARTESIAN_POINT('Ctrl Pts',(-44.6074695243589,-1.43218770176645E-14,
8.46719451744161));
#3218=CARTESIAN_POINT('Ctrl Pts',(-44.1741403300322,-1.2490009027033E-14,
8.60837654140212));
#3219=CARTESIAN_POINT('Ctrl Pts',(-43.957100425155,-9.88098491916389E-15,
8.67593604627367));
#3220=CARTESIAN_POINT('Ctrl Pts',(-43.5234563762582,-1.10467190950203E-14,
8.80511044508152));
#3221=CARTESIAN_POINT('Ctrl Pts',(-43.3066239379348,-1.48214773787458E-14,
8.86679975726875));
#3222=CARTESIAN_POINT('Ctrl Pts',(-42.6563779943798,-1.53210777398272E-14,
9.04379102211169));
#3223=CARTESIAN_POINT('Ctrl Pts',(-42.2230732679144,-1.52655665885959E-14,
9.15107362497687));
#3224=CARTESIAN_POINT('Ctrl Pts',(-41.3571906888076,-1.52655665885959E-14,
9.34749799494818));
#3225=CARTESIAN_POINT('Ctrl Pts',(-40.9245970789775,-1.53210777398272E-14,
9.43663506835774));
#3226=CARTESIAN_POINT('Ctrl Pts',(-39.6281635689816,-1.39332989590457E-14,
9.68122246026781));
#3227=CARTESIAN_POINT('Ctrl Pts',(-38.7656553292243,-1.33226762955019E-14,
9.81390977310064));
#3228=CARTESIAN_POINT('Ctrl Pts',(-37.4754796214115,-1.33226762955019E-14,
9.98225882431641));
#3229=CARTESIAN_POINT('Ctrl Pts',(-37.0460144673576,-1.47104550762833E-14,
10.0332224910664));
#3230=CARTESIAN_POINT('Ctrl Pts',(-36.188424525307,-1.52655665885959E-14,
10.1270230508065));
#3231=CARTESIAN_POINT('Ctrl Pts',(-35.7602421886007,-1.49880108324396E-14,
10.1698763527029));
#3232=CARTESIAN_POINT('Ctrl Pts',(-34.9056083623748,-1.51545442861334E-14,
10.2494008139146));
#3233=CARTESIAN_POINT('Ctrl Pts',(-34.4788493666452,-1.52655665885959E-14,
10.2862947402486));
#3234=CARTESIAN_POINT('Ctrl Pts',(-33.6238677315729,-1.52655665885959E-14,
10.3548750069945));
#3235=CARTESIAN_POINT('Ctrl Pts',(-33.1961718222826,-1.52655665885959E-14,
10.3864537666074));
#3236=CARTESIAN_POINT('Ctrl Pts',(-31.9117882640685,-1.55431223447522E-14,
10.4731744098343));
#3237=CARTESIAN_POINT('Ctrl Pts',(-31.0542758170156,-1.51545442861334E-14,
10.5202135306195));
#3238=CARTESIAN_POINT('Ctrl Pts',(-29.3366002909415,-1.4432899320127E-14,
10.5927376485604));
#3239=CARTESIAN_POINT('Ctrl Pts',(-28.4761608671941,-1.49880108324396E-14,
10.6182195605205));
#3240=CARTESIAN_POINT('Ctrl Pts',(-26.7537363343169,-1.49880108324396E-14,
10.6475149919468));
#3241=CARTESIAN_POINT('Ctrl Pts',(-25.8929997326651,-1.50990331349021E-14,
10.6513180682083));
#3242=CARTESIAN_POINT('Ctrl Pts',(-24.1717820662198,-1.52655665885959E-14,
10.6373685795577));
#3243=CARTESIAN_POINT('Ctrl Pts',(-23.3114174177265,-1.55431223447522E-14,
10.619614411021));
#3244=CARTESIAN_POINT('Ctrl Pts',(-21.5911791490513,-1.47104550762833E-14,
10.5626390207657));
#3245=CARTESIAN_POINT('Ctrl Pts',(-20.7314512337837,-1.45439216225896E-14,
10.5234146492955));
#3246=CARTESIAN_POINT('Ctrl Pts',(-19.4417924804905,-1.52655665885959E-14,
10.4485318669319));
#3247=CARTESIAN_POINT('Ctrl Pts',(-19.0122168333525,-1.53210777398272E-14,
10.4208622983205));
#3248=CARTESIAN_POINT('Ctrl Pts',(-18.1544474369902,-1.28785870856518E-14,
10.3606452684977));
#3249=CARTESIAN_POINT('Ctrl Pts',(-17.7260787333555,-9.6034291630076E-15,
10.3280962329425));
#3250=CARTESIAN_POINT('Ctrl Pts',(-16.4427007962872,-1.16018306073329E-14,
10.2239312028492));
#3251=CARTESIAN_POINT('Ctrl Pts',(-15.5892294662238,-1.52655665885959E-14,
10.1457967780066));
#3252=CARTESIAN_POINT('Ctrl Pts',(-13.0347334107054,-1.47104550762833E-14,
9.89168964726816));
#3253=CARTESIAN_POINT('Ctrl Pts',(-11.3394546576359,-1.53210777398272E-14,
9.69607640520465));
#3254=CARTESIAN_POINT('Ctrl Pts',(-7.96064496793785,-1.46549439250521E-14,
9.28568442648744));
#3255=CARTESIAN_POINT('Ctrl Pts',(-6.27708213802847,-1.33781874467331E-14,
9.07095521078264));
#3256=CARTESIAN_POINT('Ctrl Pts',(-3.75757592845614,-1.40443212615082E-14,
8.75811925740311));
#3257=CARTESIAN_POINT('Ctrl Pts',(-2.91870135734488,-1.49880108324396E-14,
8.65537011020776));
#3258=CARTESIAN_POINT('Ctrl Pts',(-1.24247939398972,-1.53210777398272E-14,
8.456625736016));
#3259=CARTESIAN_POINT('Ctrl Pts',(-0.40523588459794,-1.55431223447522E-14,
8.36067304622072));
#3260=CARTESIAN_POINT('Ctrl Pts',(0.850126830267879,-1.52655665885959E-14,
8.22432478760327));
#3261=CARTESIAN_POINT('Ctrl Pts',(1.26837589519449,-1.46549439250521E-14,
8.18020417904461));
#3262=CARTESIAN_POINT('Ctrl Pts',(2.10462556977151,-1.53210777398272E-14,
8.09488104961065));
#3263=CARTESIAN_POINT('Ctrl Pts',(2.52277657874592,-1.52655665885959E-14,
8.05377185277432));
#3264=CARTESIAN_POINT('Ctrl Pts',(3.77964787852141,-1.47104550762833E-14,
7.9342744779821));
#3265=CARTESIAN_POINT('Ctrl Pts',(4.61982937965303,-1.49880108324396E-14,
7.85932056880712));
#3266=CARTESIAN_POINT('Ctrl Pts',(6.30419335006199,-1.53210777398272E-14,
7.71319367407381));
#3267=CARTESIAN_POINT('Ctrl Pts',(7.14835445371892,-1.53210777398272E-14,
7.64197271158988));
#3268=CARTESIAN_POINT('Ctrl Pts',(8.84012615676403,-1.49324996812084E-14,
7.49709237947704));
#3269=CARTESIAN_POINT('Ctrl Pts',(9.68774962954449,-1.52655665885959E-14,
7.42345015929489));
#3270=CARTESIAN_POINT('Ctrl Pts',(11.3860360205753,-1.50990331349021E-14,
7.2672442573381));
#3271=CARTESIAN_POINT('Ctrl Pts',(12.2368316890249,-1.51545442861334E-14,
7.18468982285689));
#3272=CARTESIAN_POINT('Ctrl Pts',(13.9406285449295,-1.49880108324396E-14,
7.0034685113226));
#3273=CARTESIAN_POINT('Ctrl Pts',(14.7936901482575,-1.53210777398272E-14,
6.90483054595407));
#3274=CARTESIAN_POINT('Ctrl Pts',(16.0747466690875,-1.48214773787458E-14,
6.73844149943281));
#3275=CARTESIAN_POINT('Ctrl Pts',(16.50201152176,-1.51545442861334E-14,
6.67990037484624));
#3276=CARTESIAN_POINT('Ctrl Pts',(17.3570006606566,-1.49880108324396E-14,
6.5554161693539));
#3277=CARTESIAN_POINT('Ctrl Pts',(17.7847249958247,-1.47104550762833E-14,
6.48947667417001));
#3278=CARTESIAN_POINT('Ctrl Pts',(18.4266366353337,-1.52655665885959E-14,
6.38397561990512));
#3279=CARTESIAN_POINT('Ctrl Pts',(18.6406614273411,-1.55431223447522E-14,
6.34770897366403));
#3280=CARTESIAN_POINT('Ctrl Pts',(18.9617779205806,-1.52655665885959E-14,
6.29151504371349));
#3281=CARTESIAN_POINT('Ctrl Pts',(19.068829972339,-1.55986334959835E-14,
6.27248467831306));
#3282=CARTESIAN_POINT('Ctrl Pts',(19.2829601978757,-1.42663658664332E-14,
6.23380050962898));
#3283=CARTESIAN_POINT('Ctrl Pts',(19.3900589556033,-1.50990331349021E-14,
6.21414596127395));
#3284=CARTESIAN_POINT('Ctrl Pts',(19.6041999526691,-1.51545442861334E-14,
6.17419022140595));
#3285=CARTESIAN_POINT('Ctrl Pts',(19.7112453138705,-1.52655665885959E-14,
6.1539249037101));
#3286=CARTESIAN_POINT('Ctrl Pts',(19.927225613168,-1.52655665885959E-14,
6.11216350959792));
#3287=CARTESIAN_POINT('Ctrl Pts',(20.0357720315265,-1.52655665885959E-14,
6.09072507683146));
#3288=CARTESIAN_POINT('Ctrl Pts',(20.3635135134148,-1.52655665885959E-14,
6.02409147505319));
#3289=CARTESIAN_POINT('Ctrl Pts',(20.5844252421794,-1.49880108324396E-14,
5.97663273062336));
#3290=CARTESIAN_POINT('Ctrl Pts',(21.0302529664136,-1.51545442861334E-14,
5.87252956963633));
#3291=CARTESIAN_POINT('Ctrl Pts',(21.255123956843,-1.52655665885959E-14,
5.8158636933129));
#3292=CARTESIAN_POINT('Ctrl Pts',(21.7069290696632,-1.52655665885959E-14,
5.69053907719101));
#3293=CARTESIAN_POINT('Ctrl Pts',(21.9338427022935,-1.52655665885959E-14,
5.62185435786818));
#3294=CARTESIAN_POINT('Ctrl Pts',(22.2017782898667,-1.52655665885959E-14,
5.53241479386655));
#3295=CARTESIAN_POINT('Ctrl Pts',(22.2429910739314,-1.52655665885959E-14,
5.51842350402865));
#3296=CARTESIAN_POINT('Ctrl Pts',(22.2841887200099,-1.50990331349021E-14,
5.50419830661928));
#3297=CARTESIAN_POINT('Origin',(22.5271211105952,0.,5.95690952216869));
#3298=CARTESIAN_POINT('Ctrl Pts',(21.5644964972421,1.49999999933821,4.16303199033283));
#3299=CARTESIAN_POINT('Ctrl Pts',(21.681228802004,1.25717622640274,4.38056586163327));
#3300=CARTESIAN_POINT('Ctrl Pts',(21.7980931140595,1.01382299981494,4.59834573216322));
#3301=CARTESIAN_POINT('Ctrl Pts',(22.0379173769264,0.513975656786509,5.0452648642717));
#3302=CARTESIAN_POINT('Ctrl Pts',(22.1612401129227,0.256699533297706,5.27508018605377));
#3303=CARTESIAN_POINT('Ctrl Pts',(22.2841887197601,-1.05214455203839E-9,
5.50419830781864));
#3304=CARTESIAN_POINT('',(21.3356435067856,0.,3.73655812712738));
#3305=CARTESIAN_POINT('Origin',(21.3356435067856,0.,3.73655812712738));
#3306=CARTESIAN_POINT('Ctrl Pts',(-53.4855959126572,1.50000424468862,0.840085176636737));
#3307=CARTESIAN_POINT('Ctrl Pts',(-53.1643320247582,1.50000424468862,1.1268400488604));
#3308=CARTESIAN_POINT('Ctrl Pts',(-52.8430681368593,1.50000424468862,1.41359492108406));
#3309=CARTESIAN_POINT('Ctrl Pts',(-52.3611723050108,1.50000424468862,1.84372722941957));
#3310=CARTESIAN_POINT('Ctrl Pts',(-52.2005403610613,1.50000424468862,1.98710466553139));
#3311=CARTESIAN_POINT('Ctrl Pts',(-51.8792764731623,1.50000424468862,2.27385953775507));
#3312=CARTESIAN_POINT('Ctrl Pts',(-51.7186445292128,1.50000424468862,2.41723697386691));
#3313=CARTESIAN_POINT('Ctrl Pts',(-51.4776966132886,1.50000424468862,2.63230312803465));
#3314=CARTESIAN_POINT('Ctrl Pts',(-51.3973806413139,1.50000424468862,2.70399184609058));
#3315=CARTESIAN_POINT('Ctrl Pts',(-51.2367486973644,1.50000424468862,2.84736928220241));
#3316=CARTESIAN_POINT('Ctrl Pts',(-51.1564327253896,1.50000424468862,2.91905800025832));
#3317=CARTESIAN_POINT('Ctrl Pts',(-50.9958007814402,1.50000424468862,3.06243543637014));
#3318=CARTESIAN_POINT('Ctrl Pts',(-50.9155056164988,1.50000424468862,3.13414750105302));
#3319=CARTESIAN_POINT('Ctrl Pts',(-50.8150846427386,1.50000424468862,3.22372921533924));
#3320=CARTESIAN_POINT('Ctrl Pts',(-50.7950108515033,1.50000424468862,3.24165723150992));
#3321=CARTESIAN_POINT('Ctrl Pts',(-50.7648923620128,1.50000424468862,3.26854050078091));
#3322=CARTESIAN_POINT('Ctrl Pts',(-50.7548528655159,1.50000424468862,3.2775015905379));
#3323=CARTESIAN_POINT('Ctrl Pts',(-50.7347738725222,1.50000424468862,3.29542377005189));
#3324=CARTESIAN_POINT('Ctrl Pts',(-50.7247343760254,1.50000424468862,3.30438485980889));
#3325=CARTESIAN_POINT('Ctrl Pts',(-50.7096751312801,1.50000424468862,3.31782649444435));
#3326=CARTESIAN_POINT('Ctrl Pts',(-50.7046553830317,1.50000424468862,3.32230703932284));
#3327=CARTESIAN_POINT('Ctrl Pts',(-50.6946158865349,1.50000424468862,3.33126812907983));
#3328=CARTESIAN_POINT('Ctrl Pts',(-50.6895959364334,1.50000424468862,3.33574844718509));
#3329=CARTESIAN_POINT('Ctrl Pts',(-50.6795568436426,1.50000424468862,3.34470999048859));
#3330=CARTESIAN_POINT('Ctrl Pts',(-50.6745359674055,1.50000424468862,3.34918926458991));
#3331=CARTESIAN_POINT('Ctrl Pts',(-50.6644875302798,1.50000424468862,3.35814031000442));
#3332=CARTESIAN_POINT('Ctrl Pts',(-50.6594607930231,1.50000424468862,3.36261300364892));
#3333=CARTESIAN_POINT('Ctrl Pts',(-50.6443721387661,1.50000424468862,3.37602160585764));
#3334=CARTESIAN_POINT('Ctrl Pts',(-50.6343023847501,1.50000424468862,3.38494871278844));
#3335=CARTESIAN_POINT('Ctrl Pts',(-50.6141412499045,1.50000424468862,3.40277864154937));
#3336=CARTESIAN_POINT('Ctrl Pts',(-50.60404992209,1.50000424468862,3.41168152263516));
#3337=CARTESIAN_POINT('Ctrl Pts',(-50.5737436481473,1.50000424468863,3.43835390553867));
#3338=CARTESIAN_POINT('Ctrl Pts',(-50.5534964114456,1.50000424468862,3.45608714691913));
#3339=CARTESIAN_POINT('Ctrl Pts',(-50.5129157820777,1.50000424468862,3.49145688153963));
#3340=CARTESIAN_POINT('Ctrl Pts',(-50.4925823894169,1.50000424468862,3.50909337478607));
#3341=CARTESIAN_POINT('Ctrl Pts',(-50.4314529095512,1.50000424468862,3.56185765602773));
#3342=CARTESIAN_POINT('Ctrl Pts',(-50.3905275193144,1.50000424468862,3.59684024423588));
#3343=CARTESIAN_POINT('Ctrl Pts',(-50.2672336401988,1.50000424468862,3.70120665243317));
#3344=CARTESIAN_POINT('Ctrl Pts',(-50.1843379300463,1.50000424468862,3.77001650401763));
#3345=CARTESIAN_POINT('Ctrl Pts',(-50.0172017432821,1.50000424468862,3.90605383105355));
#3346=CARTESIAN_POINT('Ctrl Pts',(-49.9328682048228,1.50000424468862,3.97335380373027));
#3347=CARTESIAN_POINT('Ctrl Pts',(-49.7631459041653,1.50000424468862,4.10614308134383));
#3348=CARTESIAN_POINT('Ctrl Pts',(-49.677825339688,1.50000424468862,4.1715858145101));
#3349=CARTESIAN_POINT('Ctrl Pts',(-49.2487341885864,1.50000424468862,4.49422615931033));
#3350=CARTESIAN_POINT('Ctrl Pts',(-48.8978315305851,1.50000424468862,4.73757809459553));
#3351=CARTESIAN_POINT('Ctrl Pts',(-48.1815619571434,1.50000424468862,5.19646908789177));
#3352=CARTESIAN_POINT('Ctrl Pts',(-47.8162114076662,1.50000424468862,5.41201043441217));
#3353=CARTESIAN_POINT('Ctrl Pts',(-47.0720114983415,1.50000424468862,5.81708209356818));
#3354=CARTESIAN_POINT('Ctrl Pts',(-46.6931626858749,1.50000424468862,6.00661346095856));
#3355=CARTESIAN_POINT('Ctrl Pts',(-45.9229326124668,1.50000424468862,6.361527261268));
#3356=CARTESIAN_POINT('Ctrl Pts',(-45.5315517688313,1.50000424468862,6.52691049828853));
#3357=CARTESIAN_POINT('Ctrl Pts',(-44.9358235836156,1.50000424468862,6.7583042272479));
#3358=CARTESIAN_POINT('Ctrl Pts',(-44.7358048778714,1.50000424468862,6.8326556215113));
#3359=CARTESIAN_POINT('Ctrl Pts',(-44.3330075021904,1.50000424468862,6.97604020093496));
#3360=CARTESIAN_POINT('Ctrl Pts',(-44.1303004124773,1.50000424468862,7.04504995476646));
#3361=CARTESIAN_POINT('Ctrl Pts',(-43.7219662840761,1.50000424468862,7.17808841752429));
#3362=CARTESIAN_POINT('Ctrl Pts',(-43.5170844940724,1.50000424468862,7.24186840105371));
#3363=CARTESIAN_POINT('Ctrl Pts',(-43.107010875435,1.50000424468862,7.36402161595204));
#3364=CARTESIAN_POINT('Ctrl Pts',(-42.9016041135959,1.50000424468862,7.42246492070205));
#3365=CARTESIAN_POINT('Ctrl Pts',(-42.2845508414699,1.50000424468862,7.59042137367504));
#3366=CARTESIAN_POINT('Ctrl Pts',(-41.8719366383669,1.50000424468862,7.69261310357766));
#3367=CARTESIAN_POINT('Ctrl Pts',(-41.0446440327223,1.50000424468862,7.88028330663815));
#3368=CARTESIAN_POINT('Ctrl Pts',(-40.6299533000686,1.50000424468862,7.96575790042277));
#3369=CARTESIAN_POINT('Ctrl Pts',(-39.3832305879684,1.50000424468862,8.20096473155133));
#3370=CARTESIAN_POINT('Ctrl Pts',(-38.5485529379463,1.50000424468862,8.32951876556412));
#3371=CARTESIAN_POINT('Ctrl Pts',(-37.2929149715664,1.50000424468862,8.49336037753108));
#3372=CARTESIAN_POINT('Ctrl Pts',(-36.8737616841785,1.50000424468862,8.54311292039738));
#3373=CARTESIAN_POINT('Ctrl Pts',(-36.0344921391938,1.50000424468862,8.63490959633655));
#3374=CARTESIAN_POINT('Ctrl Pts',(-35.6143772910846,1.50000424468862,8.67696500794892));
#3375=CARTESIAN_POINT('Ctrl Pts',(-34.7734157326484,1.50000424468862,8.75521742500524));
#3376=CARTESIAN_POINT('Ctrl Pts',(-34.3525922942412,1.50000424468862,8.79160070265665));
#3377=CARTESIAN_POINT('Ctrl Pts',(-33.510295192155,1.50000424468862,8.85916226730201));
#3378=CARTESIAN_POINT('Ctrl Pts',(-33.0888144051685,1.50000424468862,8.89028354208506));
#3379=CARTESIAN_POINT('Ctrl Pts',(-31.8233820850184,1.50000424468862,8.97572285277626));
#3380=CARTESIAN_POINT('Ctrl Pts',(-30.9784103501772,1.50000424468862,9.02207604912839));
#3381=CARTESIAN_POINT('Ctrl Pts',(-29.2859136426566,1.50000424468862,9.09353706128219));
#3382=CARTESIAN_POINT('Ctrl Pts',(-28.4380681793794,1.50000424468862,9.11864626001917));
#3383=CARTESIAN_POINT('Ctrl Pts',(-26.7408102190484,1.50000424468862,9.14751365292547));
#3384=CARTESIAN_POINT('Ctrl Pts',(-25.8926280014397,1.50000424468862,9.15126154992858));
#3385=CARTESIAN_POINT('Ctrl Pts',(-24.196466356748,1.50000424468862,9.13751512655564));
#3386=CARTESIAN_POINT('Ctrl Pts',(-23.3486016456246,1.50000424468862,9.12001922212186));
#3387=CARTESIAN_POINT('Ctrl Pts',(-21.6533026593848,1.50000424468862,9.06386983730065));
#3388=CARTESIAN_POINT('Ctrl Pts',(-20.8059333011263,1.50000424468862,9.02520867128565));
#3389=CARTESIAN_POINT('Ctrl Pts',(-19.5350064906316,1.50000424468862,8.95141355489978));
#3390=CARTESIAN_POINT('Ctrl Pts',(-19.1115305199824,1.50000424468862,8.92413823918045));
#3391=CARTESIAN_POINT('Ctrl Pts',(-18.2652153631114,1.50000424468862,8.8647255713046));
#3392=CARTESIAN_POINT('Ctrl Pts',(-17.8422984792913,1.50000424468862,8.83259214057113));
#3393=CARTESIAN_POINT('Ctrl Pts',(-16.5743006753995,1.50000424468862,8.72967574504789));
#3394=CARTESIAN_POINT('Ctrl Pts',(-15.72988800375,1.50000424468862,8.65238116375449));
#3395=CARTESIAN_POINT('Ctrl Pts',(-13.198843265656,1.50000424468862,8.40060735977158));
#3396=CARTESIAN_POINT('Ctrl Pts',(-11.5143241645176,1.50000424468862,8.20628809518815));
#3397=CARTESIAN_POINT('Ctrl Pts',(-8.1474934174154,1.50000424468862,7.79735066775273));
#3398=CARTESIAN_POINT('Ctrl Pts',(-6.46516732482365,1.50000424468862,7.58278618092267));
#3399=CARTESIAN_POINT('Ctrl Pts',(-3.94077394457453,1.50000424468862,7.26934320881284));
#3400=CARTESIAN_POINT('Ctrl Pts',(-3.09914796278127,1.50000424468862,7.16625406252897));
#3401=CARTESIAN_POINT('Ctrl Pts',(-1.41525996229401,1.50000424468862,6.96660071619449));
#3402=CARTESIAN_POINT('Ctrl Pts',(-0.572995336836428,1.50000424468862,6.87006947964638));
#3403=CARTESIAN_POINT('Ctrl Pts',(0.691132836996335,1.50000424468862,6.73276694004229));
#3404=CARTESIAN_POINT('Ctrl Pts',(1.11263597424435,1.50000424468862,6.6883027790284));
#3405=CARTESIAN_POINT('Ctrl Pts',(1.95592373084958,1.50000424468862,6.60226135719316));
#3406=CARTESIAN_POINT('Ctrl Pts',(2.37771906724245,1.50000424468862,6.56079404822635));
#3407=CARTESIAN_POINT('Ctrl Pts',(3.64350089097926,1.50000424468862,6.44045159867955));
#3408=CARTESIAN_POINT('Ctrl Pts',(4.48783416472058,1.50000424468862,6.3651333228694));
#3409=CARTESIAN_POINT('Ctrl Pts',(6.17690063171921,1.50000424468862,6.21859844147724));
#3410=CARTESIAN_POINT('Ctrl Pts',(7.02162882253013,1.50000424468862,6.14733057126028));
#3411=CARTESIAN_POINT('Ctrl Pts',(8.71087766779818,1.50000424468862,6.0026664064732));
#3412=CARTESIAN_POINT('Ctrl Pts',(9.55541256297313,1.50000424468862,5.92928624336249));
#3413=CARTESIAN_POINT('Ctrl Pts',(11.2436012924755,1.50000424468862,5.77400940558164));
#3414=CARTESIAN_POINT('Ctrl Pts',(12.0873886915773,1.50000424468862,5.69211951289022));
#3415=CARTESIAN_POINT('Ctrl Pts',(13.7727791084152,1.50000424468862,5.51285655268981));
#3416=CARTESIAN_POINT('Ctrl Pts',(14.6144462244022,1.50000424468862,5.41550723650472));
#3417=CARTESIAN_POINT('Ctrl Pts',(15.8745706893567,1.50000424468862,5.2518376377522));
#3418=CARTESIAN_POINT('Ctrl Pts',(16.2942164913156,1.50000424468862,5.194334903692));
#3419=CARTESIAN_POINT('Ctrl Pts',(17.1325605534117,1.50000424468862,5.07227422446284));
#3420=CARTESIAN_POINT('Ctrl Pts',(17.5512592043762,1.50000424468862,5.00771918949975));
#3421=CARTESIAN_POINT('Ctrl Pts',(18.1784675269534,1.50000424468862,4.9046347381739));
#3422=CARTESIAN_POINT('Ctrl Pts',(18.3873969138115,1.50000424468862,4.86923043909388));
#3423=CARTESIAN_POINT('Ctrl Pts',(18.7005631843819,1.50000424468862,4.81442776426905));
#3424=CARTESIAN_POINT('Ctrl Pts',(18.8049139660963,1.50000424468862,4.79587744987488));
#3425=CARTESIAN_POINT('Ctrl Pts',(19.0135364870674,1.50000424468862,4.75818828779729));
#3426=CARTESIAN_POINT('Ctrl Pts',(19.1178090657383,1.50000424468862,4.73905213336367));
#3427=CARTESIAN_POINT('Ctrl Pts',(19.3262686371032,1.50000424468862,4.70015679239322));
#3428=CARTESIAN_POINT('Ctrl Pts',(19.430418771527,1.50000424468862,4.68043767856379));
#3429=CARTESIAN_POINT('Ctrl Pts',(19.6384865349788,1.50000424468862,4.64020578699138));
#3430=CARTESIAN_POINT('Ctrl Pts',(19.7424000925144,1.50000424468862,4.61967928244251));
#3431=CARTESIAN_POINT('Ctrl Pts',(20.0536422980033,1.50000424468862,4.55639894428754));
#3432=CARTESIAN_POINT('Ctrl Pts',(20.2604666189451,1.50000424468862,4.5119242877194));
#3433=CARTESIAN_POINT('Ctrl Pts',(20.6720192733516,1.50000424468862,4.41582318750738));
#3434=CARTESIAN_POINT('Ctrl Pts',(20.876742698695,1.50000424468862,4.36417999658545));
#3435=CARTESIAN_POINT('Ctrl Pts',(21.2834003998586,1.50000424468862,4.25137663415474));
#3436=CARTESIAN_POINT('Ctrl Pts',(21.4853308265756,1.50000424468862,4.19020332993022));
#3437=CARTESIAN_POINT('Ctrl Pts',(21.8858633741466,1.50000424468862,4.05650003242997));
#3438=CARTESIAN_POINT('Ctrl Pts',(22.0844642714823,1.50000424468862,3.98396462045235));
#3439=CARTESIAN_POINT('Ctrl Pts',(22.4780037152932,1.50000424468862,3.82640225072584));
#3440=CARTESIAN_POINT('Ctrl Pts',(22.6729727572114,1.50000424468862,3.74136495201728));
#3441=CARTESIAN_POINT('Ctrl Pts',(22.9625022501059,1.50000424468862,3.60416799032947));
#3442=CARTESIAN_POINT('Ctrl Pts',(23.0582039529822,1.50000424468862,3.55698868386574));
#3443=CARTESIAN_POINT('Ctrl Pts',(23.2480654317315,1.50000424468862,3.45977570935616));
#3444=CARTESIAN_POINT('Ctrl Pts',(23.3422185562957,1.50000424468862,3.40974593973871));
#3445=CARTESIAN_POINT('Ctrl Pts',(23.48231624516,1.50000424468862,3.33262936836403));
#3446=CARTESIAN_POINT('Ctrl Pts',(23.5288269086232,1.50000424468862,3.30657870843009));
#3447=CARTESIAN_POINT('Ctrl Pts',(23.6214777127621,1.50000424468862,3.25379921372457));
#3448=CARTESIAN_POINT('Ctrl Pts',(23.6676163291091,1.50000424468862,3.22706758916978));
#3449=CARTESIAN_POINT('Ctrl Pts',(23.7365562716072,1.50000424468862,3.18647965905807));
#3450=CARTESIAN_POINT('Ctrl Pts',(23.7594884622631,1.50000424468862,3.17286287905752));
#3451=CARTESIAN_POINT('Ctrl Pts',(23.805268896492,1.50000424468862,3.14547566219199));
#3452=CARTESIAN_POINT('Ctrl Pts',(23.8281202947054,1.50000424468862,3.13171099952304));
#3453=CARTESIAN_POINT('Ctrl Pts',(23.8965947007905,1.50000424468862,3.09027096277851));
#3454=CARTESIAN_POINT('Ctrl Pts',(23.9421431991977,1.50000424468862,3.06245920626797));
#3455=CARTESIAN_POINT('Ctrl Pts',(24.0787585992021,1.50000424468862,2.97896881982385));
#3456=CARTESIAN_POINT('Ctrl Pts',(24.1697954746497,1.50000424468862,2.92323520931005));
#3457=CARTESIAN_POINT('Ctrl Pts',(24.3529430457551,1.50000424468862,2.81373335788034));
#3458=CARTESIAN_POINT('Ctrl Pts',(24.4450438892746,1.50000424468862,2.75993301037979));
#3459=CARTESIAN_POINT('Ctrl Pts',(24.7244481055146,1.50000424468862,2.60429339584203));
#3460=CARTESIAN_POINT('Ctrl Pts',(24.9149058159532,1.50000424468862,2.50796758924331));
#3461=CARTESIAN_POINT('Ctrl Pts',(25.1135772365769,1.50000424468862,2.4271963168569));
#3462=CARTESIAN_POINT('Ctrl Pts',(-54.4844548707889,-4.24468864876006E-6,
1.95915007643658));
#3463=CARTESIAN_POINT('Ctrl Pts',(-54.1631909828898,-4.24468864876006E-6,
2.24590494866024));
#3464=CARTESIAN_POINT('Ctrl Pts',(-53.8419270949909,-4.24468864876006E-6,
2.5326598208839));
#3465=CARTESIAN_POINT('Ctrl Pts',(-53.3600312631424,-4.24468864876006E-6,
2.96279212921941));
#3466=CARTESIAN_POINT('Ctrl Pts',(-53.199399319193,-4.24468864876006E-6,
3.10616956533124));
#3467=CARTESIAN_POINT('Ctrl Pts',(-52.878135431294,-4.24468864876006E-6,
3.39292443755491));
#3468=CARTESIAN_POINT('Ctrl Pts',(-52.7175034873445,-4.24468864876006E-6,
3.53630187366676));
#3469=CARTESIAN_POINT('Ctrl Pts',(-52.4765555714202,-4.24468864876006E-6,
3.75136802783449));
#3470=CARTESIAN_POINT('Ctrl Pts',(-52.3962395994455,-4.24468864876006E-6,
3.82305674589042));
#3471=CARTESIAN_POINT('Ctrl Pts',(-52.235607655496,-4.24468864876006E-6,
3.96643418200225));
#3472=CARTESIAN_POINT('Ctrl Pts',(-52.1552916835213,-4.24468864876006E-6,
4.03812290005816));
#3473=CARTESIAN_POINT('Ctrl Pts',(-51.9946597395718,-4.24468864876006E-6,
4.18150033616999));
#3474=CARTESIAN_POINT('Ctrl Pts',(-51.9144227402979,-4.24468864876006E-6,
4.25316422926206));
#3475=CARTESIAN_POINT('Ctrl Pts',(-51.8139290594534,-4.24468864876006E-6,
4.34280615803678));
#3476=CARTESIAN_POINT('Ctrl Pts',(-51.793869809635,-4.24468864876006E-6,
4.36072213130976));
#3477=CARTESIAN_POINT('Ctrl Pts',(-51.7637513201444,-4.24468864876006E-6,
4.38760540058075));
#3478=CARTESIAN_POINT('Ctrl Pts',(-51.7537118236476,-4.24468864876006E-6,
4.39656649033775));
#3479=CARTESIAN_POINT('Ctrl Pts',(-51.7336328306539,-4.24468864876006E-6,
4.41448866985173));
#3480=CARTESIAN_POINT('Ctrl Pts',(-51.723593334157,-4.24468864876006E-6,
4.42344975960873));
#3481=CARTESIAN_POINT('Ctrl Pts',(-51.7085340894118,-4.24468864876006E-6,
4.43689139424419));
#3482=CARTESIAN_POINT('Ctrl Pts',(-51.7035143411634,-4.24468864876006E-6,
4.44137193912269));
#3483=CARTESIAN_POINT('Ctrl Pts',(-51.6934748446665,-4.24468864876006E-6,
4.45033302887968));
#3484=CARTESIAN_POINT('Ctrl Pts',(-51.688438436341,-4.24468864876006E-6,
4.45482800098852));
#3485=CARTESIAN_POINT('Ctrl Pts',(-51.6784322599983,-4.24468864876006E-6,
4.46376023628484));
#3486=CARTESIAN_POINT('Ctrl Pts',(-51.6726924455922,-4.24468864919374E-6,
4.46888101943176));
#3487=CARTESIAN_POINT('Ctrl Pts',(-51.6618473995543,-4.24468864832638E-6,
4.47854149516085));
#3488=CARTESIAN_POINT('Ctrl Pts',(-51.6562970666484,-4.24468864876006E-6,
4.4834802833282));
#3489=CARTESIAN_POINT('Ctrl Pts',(-51.6399334159774,-4.24468864919374E-6,
4.49802163123191));
#3490=CARTESIAN_POINT('Ctrl Pts',(-51.6289156084215,-4.2446886500611E-6,
4.50778950698426));
#3491=CARTESIAN_POINT('Ctrl Pts',(-51.606953166536,-4.2446886500611E-6,
4.52721245996945));
#3492=CARTESIAN_POINT('Ctrl Pts',(-51.5959601033195,-4.24468864919374E-6,
4.53691088012528));
#3493=CARTESIAN_POINT('Ctrl Pts',(-51.5629454085781,-4.24468864615798E-6,
4.56596692908652));
#3494=CARTESIAN_POINT('Ctrl Pts',(-51.540888271787,-4.24468864832638E-6,
4.58528534624317));
#3495=CARTESIAN_POINT('Ctrl Pts',(-51.4966794380725,-4.24468864919374E-6,
4.62381739320071));
#3496=CARTESIAN_POINT('Ctrl Pts',(-51.4745277411724,-4.24468864876006E-6,
4.64303102300578));
#3497=CARTESIAN_POINT('Ctrl Pts',(-51.4079309999015,-4.24468864919374E-6,
4.70051440404672));
#3498=CARTESIAN_POINT('Ctrl Pts',(-51.3633443025652,-4.24468864832638E-6,
4.73862664451631));
#3499=CARTESIAN_POINT('Ctrl Pts',(-51.2290192229532,-4.2446886478927E-6,
4.85233079692795));
#3500=CARTESIAN_POINT('Ctrl Pts',(-51.1387054721567,-4.24468864919374E-6,
4.92729816849616));
#3501=CARTESIAN_POINT('Ctrl Pts',(-50.9566223990134,-4.24468864832638E-6,
5.07550122998796));
#3502=CARTESIAN_POINT('Ctrl Pts',(-50.8647517193264,-4.24468864919374E-6,
5.14881587934781));
#3503=CARTESIAN_POINT('Ctrl Pts',(-50.6798829713378,-4.24468864832638E-6,
5.29345560729514));
#3504=CARTESIAN_POINT('Ctrl Pts',(-50.5869592637586,-4.24468864876006E-6,
5.36472995902057));
#3505=CARTESIAN_POINT('Ctrl Pts',(-50.1197166576145,-4.24468864876006E-6,
5.71605669911536));
#3506=CARTESIAN_POINT('Ctrl Pts',(-49.7378925849801,-4.24468864876006E-6,
5.98082726797411));
#3507=CARTESIAN_POINT('Ctrl Pts',(-48.9598685421464,-4.24468864876006E-6,
6.47928168267429));
#3508=CARTESIAN_POINT('Ctrl Pts',(-48.563691410888,-4.24468864876006E-6,
6.71296978926406));
#3509=CARTESIAN_POINT('Ctrl Pts',(-47.7587612895418,-4.24468864876006E-6,
7.15109650890973));
#3510=CARTESIAN_POINT('Ctrl Pts',(-47.3500117097391,-4.24468864832638E-6,
7.35553976657944));
#3511=CARTESIAN_POINT('Ctrl Pts',(-46.5215827116132,-4.24468864919374E-6,
7.73727044476595));
#3512=CARTESIAN_POINT('Ctrl Pts',(-46.1019043152216,-4.24468864832638E-6,
7.91456257082263));
#3513=CARTESIAN_POINT('Ctrl Pts',(-45.4653047942148,-4.24468864876006E-6,
8.16183140099499));
#3514=CARTESIAN_POINT('Ctrl Pts',(-45.251923396063,-4.24468864876006E-6,
8.24114413294632));
#3515=CARTESIAN_POINT('Ctrl Pts',(-44.8229684642909,-4.24468864919374E-6,
8.39384005981013));
#3516=CARTESIAN_POINT('Ctrl Pts',(-44.6074708746446,-4.24468864876006E-6,
8.46719854180413));
#3517=CARTESIAN_POINT('Ctrl Pts',(-44.1741416095873,-4.24468864876006E-6,
8.60838058880916));
#3518=CARTESIAN_POINT('Ctrl Pts',(-43.9571016703052,-4.24468864876006E-6,
8.67594010437595));
#3519=CARTESIAN_POINT('Ctrl Pts',(-43.5234575547092,-4.24468864876006E-6,
8.80511452305223));
#3520=CARTESIAN_POINT('Ctrl Pts',(-43.3066250840536,-4.24468864876006E-6,
8.86680384442496));
#3521=CARTESIAN_POINT('Ctrl Pts',(-42.6563790465704,-4.24468864876006E-6,
9.04379513483447));
#3522=CARTESIAN_POINT('Ctrl Pts',(-42.2230742615554,-4.24468864876006E-6,
9.15107775210572));
#3523=CARTESIAN_POINT('Ctrl Pts',(-41.3571915732473,-4.24468864876006E-6,
9.34750214684944));
#3524=CARTESIAN_POINT('Ctrl Pts',(-40.9245979127559,-4.24468864876006E-6,
9.43663923062303));
#3525=CARTESIAN_POINT('Ctrl Pts',(-39.6281642620891,-4.24468864832638E-6,
9.68122664907806));
#3526=CARTESIAN_POINT('Ctrl Pts',(-38.7656559435773,-4.24468864876006E-6,
9.81391397360718));
#3527=CARTESIAN_POINT('Ctrl Pts',(-37.4754801380301,-4.24468864876006E-6,
9.98226303757803));
#3528=CARTESIAN_POINT('Ctrl Pts',(-37.0460149547959,-4.24468864832638E-6,
10.0332267077553));
#3529=CARTESIAN_POINT('Ctrl Pts',(-36.1884249609025,-4.24468864876006E-6,
10.1270272731659));
#3530=CARTESIAN_POINT('Ctrl Pts',(-35.760242601367,-4.24468864876006E-6,
10.1698805773202));
#3531=CARTESIAN_POINT('Ctrl Pts',(-34.9056087364515,-4.24468864876006E-6,
10.2494050421315));
#3532=CARTESIAN_POINT('Ctrl Pts',(-34.4788497239255,-4.24468864876006E-6,
10.2862989699105));
#3533=CARTESIAN_POINT('Ctrl Pts',(-33.6238680529587,-4.24468864876006E-6,
10.3548792395391));
#3534=CARTESIAN_POINT('Ctrl Pts',(-33.196172126081,-4.24468864876006E-6,
10.3864580004466));
#3535=CARTESIAN_POINT('Ctrl Pts',(-31.9117885142389,-4.24468864919374E-6,
10.4731786472994));
#3536=CARTESIAN_POINT('Ctrl Pts',(-31.0542760316985,-4.24468864876006E-6,
10.5202177700256));
#3537=CARTESIAN_POINT('Ctrl Pts',(-29.3366004343738,-4.24468864832638E-6,
10.5927418909748));
#3538=CARTESIAN_POINT('Ctrl Pts',(-28.4761609749882,-4.24468864876006E-6,
10.6182238039896));
#3539=CARTESIAN_POINT('Ctrl Pts',(-26.753736370895,-4.24468864876006E-6,
10.6475192366273));
#3540=CARTESIAN_POINT('Ctrl Pts',(-25.8929997337171,-4.24468864876006E-6,
10.6513223130449));
#3541=CARTESIAN_POINT('Ctrl Pts',(-24.1717819963686,-4.24468864876006E-6,
10.6373728238196));
#3542=CARTESIAN_POINT('Ctrl Pts',(-23.3114173125031,-4.24468864919374E-6,
10.6196186545521));
#3543=CARTESIAN_POINT('Ctrl Pts',(-21.5911789732551,-4.24468864832638E-6,
10.5626432619593));
#3544=CARTESIAN_POINT('Ctrl Pts',(-20.7314510230155,-4.24468864832638E-6,
10.5234188888955));
#3545=CARTESIAN_POINT('Ctrl Pts',(-19.441792216715,-4.24468864876006E-6,
10.448536103454));
#3546=CARTESIAN_POINT('Ctrl Pts',(-19.0122165523162,-4.24468864876006E-6,
10.4208665337269));
#3547=CARTESIAN_POINT('Ctrl Pts',(-18.1544471235408,-4.24468864876006E-6,
10.3606495016279));
#3548=CARTESIAN_POINT('Ctrl Pts',(-17.7260784044787,-4.24468864876006E-6,
10.3281004648967));
#3549=CARTESIAN_POINT('Ctrl Pts',(-16.4427004238879,-4.24468864919374E-6,
10.22393543127));
#3550=CARTESIAN_POINT('Ctrl Pts',(-15.5892290681904,-4.24468864876006E-6,
10.1458010040509));
#3551=CARTESIAN_POINT('Ctrl Pts',(-13.0347329463099,-4.24468864832638E-6,
9.89169386670957));
#3552=CARTESIAN_POINT('Ctrl Pts',(-11.3394541627929,-4.24468864876006E-6,
9.69608062098439));
#3553=CARTESIAN_POINT('Ctrl Pts',(-7.96064443919703,-4.24468864876006E-6,
9.28568863815111));
#3554=CARTESIAN_POINT('Ctrl Pts',(-6.27708160578794,-4.24468864876006E-6,
9.07095942198016));
#3555=CARTESIAN_POINT('Ctrl Pts',(-3.75757541004525,-4.24468864876006E-6,
8.75812347031837));
#3556=CARTESIAN_POINT('Ctrl Pts',(-2.91870084671988,-4.24468864876006E-6,
8.65537432408514));
#3557=CARTESIAN_POINT('Ctrl Pts',(-1.24247890505796,-4.24468864876006E-6,
8.45662995246558));
#3558=CARTESIAN_POINT('Ctrl Pts',(-0.405235409874857,-4.24468864919374E-6,
8.36067726430746));
#3559=CARTESIAN_POINT('Ctrl Pts',(0.850127280186599,-4.24468864876006E-6,
8.22432900839042));
#3560=CARTESIAN_POINT('Ctrl Pts',(1.26837633590489,-4.24468864876006E-6,
8.18020840080394));
#3561=CARTESIAN_POINT('Ctrl Pts',(2.10462599056565,-4.24468864876006E-6,
8.09488527340259));
#3562=CARTESIAN_POINT('Ctrl Pts',(2.5227769892274,-4.24468864876006E-6,
8.05377607757964));
#3563=CARTESIAN_POINT('Ctrl Pts',(3.77964826378803,-4.24468864832638E-6,
7.9342787051788));
#3564=CARTESIAN_POINT('Ctrl Pts',(4.61982975317104,-4.24468864876006E-6,
7.8593247970349));
#3565=CARTESIAN_POINT('Ctrl Pts',(6.30419371027295,-4.24468864876006E-6,
7.7131979034561));
#3566=CARTESIAN_POINT('Ctrl Pts',(7.14835481232514,-4.24468864876006E-6,
7.64197694110491));
#3567=CARTESIAN_POINT('Ctrl Pts',(8.84012652250938,-4.24468864919374E-6,
7.49709660838037));
#3568=CARTESIAN_POINT('Ctrl Pts',(9.68775000402986,-4.24468864876006E-6,
7.42345438745665));
#3569=CARTESIAN_POINT('Ctrl Pts',(11.3860364236348,-4.24468864876006E-6,
7.26724848287081));
#3570=CARTESIAN_POINT('Ctrl Pts',(12.2368321119163,-4.24468864876006E-6,
7.18469404650909));
#3571=CARTESIAN_POINT('Ctrl Pts',(13.9406290199073,-4.24468864876006E-6,
7.00347272943309));
#3572=CARTESIAN_POINT('Ctrl Pts',(14.7936906554792,-4.24468864876006E-6,
6.90483476041796));
#3573=CARTESIAN_POINT('Ctrl Pts',(16.0747472355423,-4.24468864876006E-6,
6.73844570620125));
#3574=CARTESIAN_POINT('Ctrl Pts',(16.5020121097752,-4.24468864876006E-6,
6.67990457867625));
#3575=CARTESIAN_POINT('Ctrl Pts',(17.3570012957737,-4.24468864876006E-6,
6.55542036632586));
#3576=CARTESIAN_POINT('Ctrl Pts',(17.7847256564825,-4.24468864832638E-6,
6.48948086722424));
#3577=CARTESIAN_POINT('Ctrl Pts',(18.4266373375988,-4.24468864876006E-6,
6.38397980612089));
#3578=CARTESIAN_POINT('Ctrl Pts',(18.6406621440251,-4.24468864919374E-6,
6.34771315743955));
#3579=CARTESIAN_POINT('Ctrl Pts',(18.961778659762,-4.24468864876006E-6,
6.29151922355206));
#3580=CARTESIAN_POINT('Ctrl Pts',(19.0688307191644,-4.24468864919374E-6,
6.27248885679318));
#3581=CARTESIAN_POINT('Ctrl Pts',(19.2829609602867,-4.24468864832638E-6,
6.23380468529344));
#3582=CARTESIAN_POINT('Ctrl Pts',(19.3900597260118,-4.24468864919374E-6,
6.21415013547148));
#3583=CARTESIAN_POINT('Ctrl Pts',(19.6042007391548,-4.24468864876006E-6,
6.17419439260278));
#3584=CARTESIAN_POINT('Ctrl Pts',(19.7112461085491,-4.24468864876006E-6,
6.15392907336129));
#3585=CARTESIAN_POINT('Ctrl Pts',(19.9272264302374,-4.24468864876006E-6,
6.11216767492095));
#3586=CARTESIAN_POINT('Ctrl Pts',(20.0357728617059,-4.24468864876006E-6,
6.09072923957392));
#3587=CARTESIAN_POINT('Ctrl Pts',(20.3635143902835,-4.24468864876006E-6,
6.02409562830664));
#3588=CARTESIAN_POINT('Ctrl Pts',(20.5844261589125,-4.24468864876006E-6,
5.97663687543248));
#3589=CARTESIAN_POINT('Ctrl Pts',(21.0302539801377,-4.24468864876006E-6,
5.87253369180135));
#3590=CARTESIAN_POINT('Ctrl Pts',(21.2551250275804,-4.24468864876006E-6,
5.8158678012648));
#3591=CARTESIAN_POINT('Ctrl Pts',(21.706930268158,-4.24468864876006E-6,
5.69054314971047));
#3592=CARTESIAN_POINT('Ctrl Pts',(21.9338439714855,-4.24468864876006E-6,
5.62185840913194));
#3593=CARTESIAN_POINT('Ctrl Pts',(22.3872744277703,-4.24468864876006E-6,
5.47049881303899));
#3594=CARTESIAN_POINT('Ctrl Pts',(22.6137579556259,-4.24468864876006E-6,
5.3878160953161));
#3595=CARTESIAN_POINT('Ctrl Pts',(23.0637791743541,-4.24468864876006E-6,
5.20764012428314));
#3596=CARTESIAN_POINT('Ctrl Pts',(23.2873232366555,-4.24468864919374E-6,
5.11014492079912));
#3597=CARTESIAN_POINT('Ctrl Pts',(23.6188171790401,-4.24468864876006E-6,
4.95306204865404));
#3598=CARTESIAN_POINT('Ctrl Pts',(23.7283127561718,-4.24468864876006E-6,
4.89908055545908));
#3599=CARTESIAN_POINT('Ctrl Pts',(23.9452217954513,-4.24468864876006E-6,
4.78801861755573));
#3600=CARTESIAN_POINT('Ctrl Pts',(24.052627331722,-4.24468864919374E-6,
4.73094334456363));
#3601=CARTESIAN_POINT('Ctrl Pts',(24.2121137015532,-4.24468864919374E-6,
4.64315427997084));
#3602=CARTESIAN_POINT('Ctrl Pts',(24.2650059892836,-4.24468864876006E-6,
4.6135287181131));
#3603=CARTESIAN_POINT('Ctrl Pts',(24.370247935397,-4.24468864876006E-6,
4.553576546795));
#3604=CARTESIAN_POINT('Ctrl Pts',(24.4225865320031,-4.24468864876006E-6,
4.52325171765904));
#3605=CARTESIAN_POINT('Ctrl Pts',(24.5007207602356,-4.24468864876006E-6,
4.47725157068682));
#3606=CARTESIAN_POINT('Ctrl Pts',(24.5268414243549,-4.24468864919374E-6,
4.46174045687451));
#3607=CARTESIAN_POINT('Ctrl Pts',(24.5779990494117,-4.24468864832638E-6,
4.43113607626247));
#3608=CARTESIAN_POINT('Ctrl Pts',(24.6030407728393,-4.24468864876006E-6,
4.41605091568199));
#3609=CARTESIAN_POINT('Ctrl Pts',(24.6765864688913,-4.24468864919374E-6,
4.37154031068307));
#3610=CARTESIAN_POINT('Ctrl Pts',(24.724019847109,-4.24468864876006E-6,
4.3425731441949));
#3611=CARTESIAN_POINT('Ctrl Pts',(24.8616938128042,-4.24468864876006E-6,
4.25843914221016));
#3612=CARTESIAN_POINT('Ctrl Pts',(24.9483601377191,-4.24468864876006E-6,
4.20540803699128));
#3613=CARTESIAN_POINT('Ctrl Pts',(25.1139167318624,-4.24468864876006E-6,
4.10642432159279));
#3614=CARTESIAN_POINT('Ctrl Pts',(25.1927679440333,-4.24468864876006E-6,
4.06045407352152));
#3615=CARTESIAN_POINT('Ctrl Pts',(25.4191698874029,-4.24468864876006E-6,
3.93433064558436));
#3616=CARTESIAN_POINT('Ctrl Pts',(25.5560295617271,-4.24468864876006E-6,
3.86643808531681));
#3617=CARTESIAN_POINT('Ctrl Pts',(25.6783212705344,-4.24468864876006E-6,
3.8168328320339));
#12112=UNCERTAINTY_MEASURE_WITH_UNIT(LENGTH_MEASURE(0.01),#12138,
'DISTANCE_ACCURACY_VALUE',
'Maximum model space distance between geometric entities at asserted c
onnectivities');
#12123=UNCERTAINTY_MEASURE_WITH_UNIT(LENGTH_MEASURE(0.01),#12138,
'DISTANCE_ACCURACY_VALUE',
'Maximum model space distance between geometric entities at asserted c
onnectivities');
#12126=(
GEOMETRIC_REPRESENTATION_CONTEXT(3)
GLOBAL_UNCERTAINTY_ASSIGNED_CONTEXT((#12112))
GLOBAL_UNIT_ASSIGNED_CONTEXT((#12138,#12140,#12141))
REPRESENTATION_CONTEXT('','3D')
);
#12137=(
GEOMETRIC_REPRESENTATION_CONTEXT(3)
GLOBAL_UNCERTAINTY_ASSIGNED_CONTEXT((#12123))
GLOBAL_UNIT_ASSIGNED_CONTEXT((#12138,#12140,#12141))
REPRESENTATION_CONTEXT('','3D')
);
#12138=(
LENGTH_UNIT()
NAMED_UNIT(*)
SI_UNIT(.MILLI.,.METRE.)
);
#12140=(
NAMED_UNIT(*)
PLANE_ANGLE_UNIT()
SI_UNIT($,.RADIAN.)
);
#12141=(
NAMED_UNIT(*)
SI_UNIT($,.STERADIAN.)
SOLID_ANGLE_UNIT()
);
#12144=SHAPE_DEFINITION_REPRESENTATION(#12157,#12185);
#12157=PRODUCT_DEFINITION_SHAPE('',$,#12199);
#12185=SHAPE_REPRESENTATION('',(#1997),#12126);
#12196=PRODUCT_DEFINITION_CONTEXT('part definition',#12237,'design');
#12199=PRODUCT_DEFINITION('knife','knife',#12212,#12196);
#12212=PRODUCT_DEFINITION_FORMATION('',$,#12241);
#12237=APPLICATION_CONTEXT(
'Core Data for Automotive Mechanical Design Process');
#12238=PRODUCT_CONTEXT('part definition',#12237,'mechanical');
#12241=PRODUCT('knife','knife',$,(#12238));
#12253=PRESENTATION_STYLE_ASSIGNMENT((#12255));
#12255=SURFACE_STYLE_USAGE(.BOTH.,#12257);
#12257=SURFACE_SIDE_STYLE('',(#12259));
#12259=SURFACE_STYLE_FILL_AREA(#12261);
#12261=FILL_AREA_STYLE('Opaque(23,69,131)',(#12263));
#12263=FILL_AREA_STYLE_COLOUR('Opaque(23,69,131)',#12265);
#12265=COLOUR_RGB('Opaque(23,69,131)',0.0901960784313725,0.270588235294118,
0.513725490196078);
ENDSEC;
END-ISO-10303-21;
